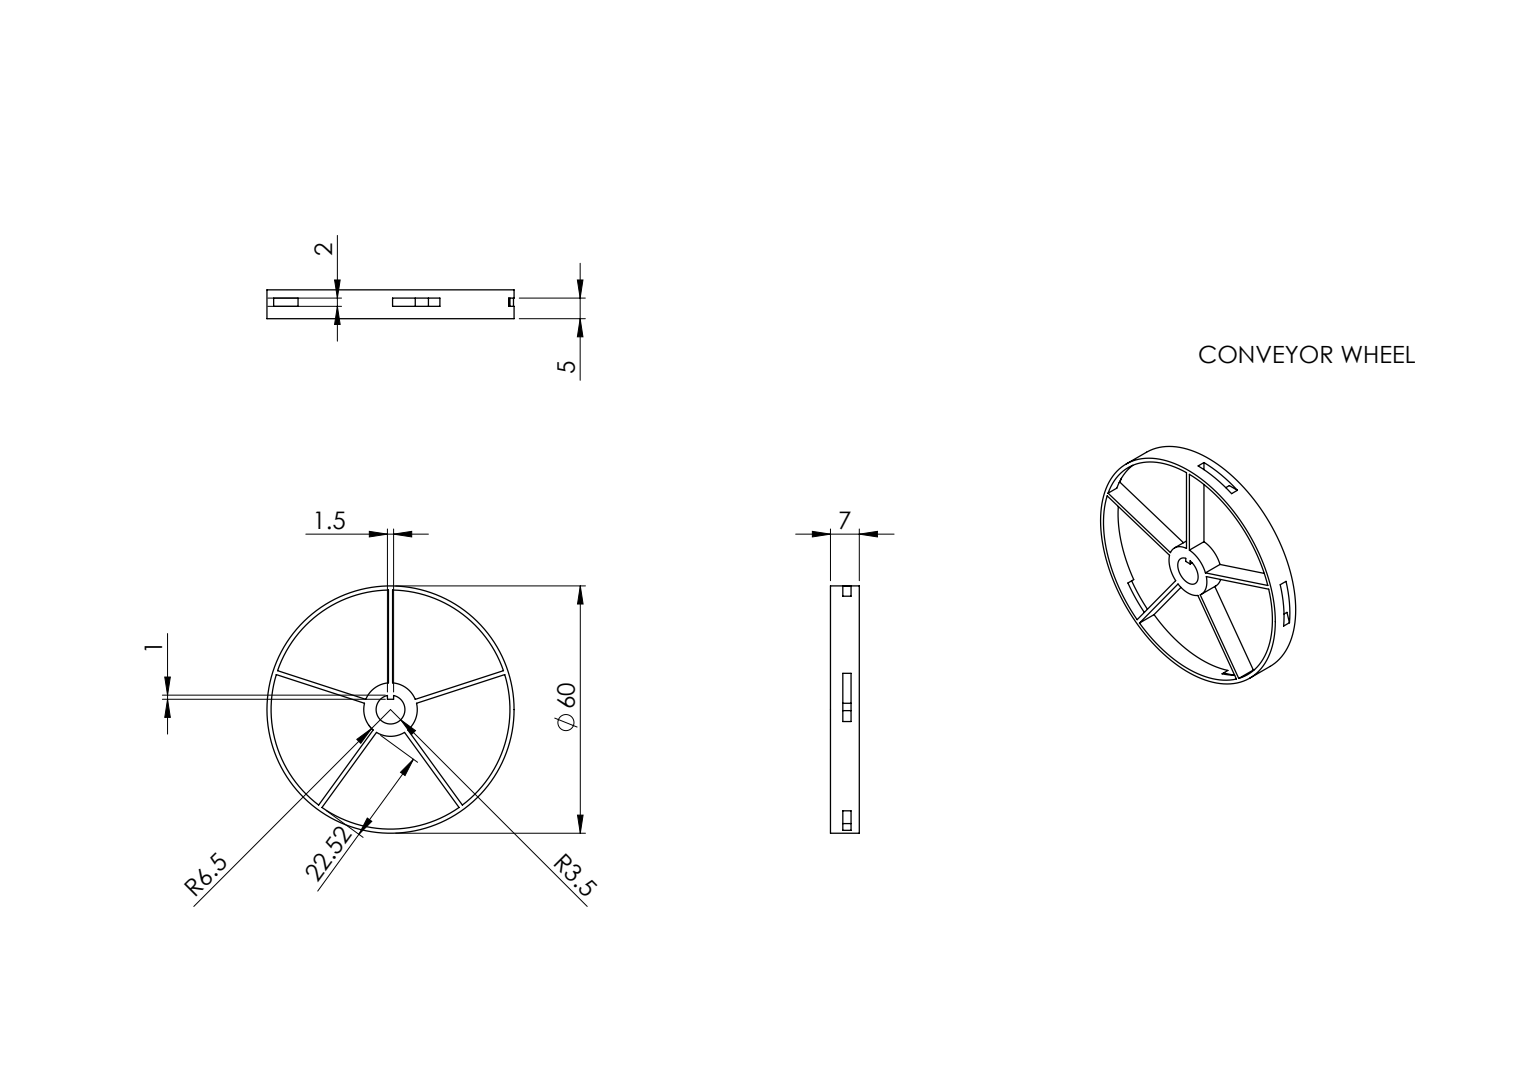
ISO-10303-21;
HEADER;
FILE_DESCRIPTION (('STEP AP214'),
    '1' );
FILE_NAME ('conveyor wheel.step',
    '2026-10-26T05:17:54',
    ( '' ),
    ( '' ),
    'SwSTEP 2.0',
    'SolidWorks 2026',
    '' );
FILE_SCHEMA (( 'AUTOMOTIVE_DESIGN' ));
ENDSEC;

DATA;
#6=FACE_OUTER_BOUND ( 'NONE', #10030, .T. ) ;
#9=CARTESIAN_POINT ( 'NONE',  ( 15.77218708916995560, 135.9950860171967975, 1.000000000000003109 ) ) ;
#22=B_SPLINE_CURVE_WITH_KNOTS ( 'NONE', 3,
 ( #4736, #8602, #10562, #11406 ),
 .UNSPECIFIED., .F., .F.,
 ( 4, 4 ),
 ( 0.000000000000000000, 0.5999999999999992006 ),
 .UNSPECIFIED. ) ;
#23=CARTESIAN_POINT ( 'NONE',  ( 65.00000000000000000, 90.00000000000000000, -3.000000000000000000 ) ) ;
#35=DIRECTION ( 'NONE',  ( -0.000000000000000000, -0.000000000000000000, -1.000000000000000000 ) ) ;
#36=VERTEX_POINT ( 'NONE', #3665 ) ;
#37=LINE ( 'NONE', #7913, #8415 ) ;
#68=ORIENTED_EDGE ( 'NONE', *, *, #7335, .T. ) ;
#69=CARTESIAN_POINT ( 'NONE',  ( 17.26299177799148055, 43.12143982588584379, 1.000000000000003109 ) ) ;
#77=VECTOR ( 'NONE', #7626, 1000.000000000000000 ) ;
#94=CIRCLE ( 'NONE', #5951, 0.9999999999999991118 ) ;
#99=ORIENTED_EDGE ( 'NONE', *, *, #9615, .F. ) ;
#111=FACE_OUTER_BOUND ( 'NONE', #2814, .T. ) ;
#133=LINE ( 'NONE', #6034, #1273 ) ;
#147=ORIENTED_EDGE ( 'NONE', *, *, #622, .F. ) ;
#155=DIRECTION ( 'NONE',  ( -1.000000000000000000, 0.000000000000000000, -0.000000000000000000 ) ) ;
#171=ORIENTED_EDGE ( 'NONE', *, *, #11272, .F. ) ;
#194=CIRCLE ( 'NONE', #6260, 3.499999999999996003 ) ;
#196=ORIENTED_EDGE ( 'NONE', *, *, #12600, .T. ) ;
#199=EDGE_LOOP ( 'NONE', ( #6657, #5220, #2552, #8518 ) ) ;
#210=VECTOR ( 'NONE', #6420, 1000.000000000000000 ) ;
#219=DIRECTION ( 'NONE',  ( 0.000000000000000000, 0.000000000000000000, -1.000000000000000000 ) ) ;
#221=ADVANCED_FACE ( 'NONE', ( #5806 ), #2080, .F. ) ;
#222=PLANE ( 'NONE',  #9692 ) ;
#229=PLANE ( 'NONE',  #10368 ) ;
#233=ORIENTED_EDGE ( 'NONE', *, *, #6025, .F. ) ;
#235=DIRECTION ( 'NONE',  ( -1.000000000000000000, 0.000000000000000000, 0.000000000000000000 ) ) ;
#238=CIRCLE ( 'NONE', #3615, 3.499999999999996003 ) ;
#239=DIRECTION ( 'NONE',  ( 0.000000000000000000, 0.000000000000000000, -1.000000000000000000 ) ) ;
#244=EDGE_CURVE ( 'NONE', #12399, #6272, #479, .T. ) ;
#260=ADVANCED_FACE ( 'NONE', ( #3129 ), #3324, .T. ) ;
#267=CARTESIAN_POINT ( 'NONE',  ( 31.59522469073171891, 84.46307801270442894, 22.38477631085024555 ) ) ;
#274=CARTESIAN_POINT ( 'NONE',  ( 44.20597631976078645, 117.5000000000000568, 4.000000000000000000 ) ) ;
#279=DIRECTION ( 'NONE',  ( -0.5877852522924753575, 0.8090169943749458970, 0.000000000000000000 ) ) ;
#284=AXIS2_PLACEMENT_3D ( 'NONE', #3967, #808, #3834 ) ;
#291=CARTESIAN_POINT ( 'NONE',  ( 35.75000000000000711, 92.49999999999998579, 4.000000000000000000 ) ) ;
#314=LINE ( 'NONE', #2362, #12520 ) ;
#321=DIRECTION ( 'NONE',  ( -0.000000000000000000, -0.000000000000000000, -1.000000000000000000 ) ) ;
#328=ORIENTED_EDGE ( 'NONE', *, *, #4950, .F. ) ;
#330=VERTEX_POINT ( 'NONE', #11158 ) ;
#331=LINE ( 'NONE', #11396, #210 ) ;
#335=ADVANCED_FACE ( 'NONE', ( #1345 ), #222, .F. ) ;
#339=DIRECTION ( 'NONE',  ( -0.5877852522924715828, -0.8090169943749484505, 0.000000000000000000 ) ) ;
#344=CARTESIAN_POINT ( 'NONE',  ( 41.31805916882746743, 91.52713075379783447, 22.38477631085024555 ) ) ;
#348=ORIENTED_EDGE ( 'NONE', *, *, #6229, .T. ) ;
#349=EDGE_CURVE ( 'NONE', #2081, #11940, #2919, .T. ) ;
#352=DIRECTION ( 'NONE',  ( -1.000000000000000000, 0.000000000000000000, 0.000000000000000000 ) ) ;
#353=CARTESIAN_POINT ( 'NONE',  ( 62.42613047537196991, 99.43702109502110886, 4.000000000000000000 ) ) ;
#354=CARTESIAN_POINT ( 'NONE',  ( 17.55170909815984004, 66.83416404266884570, 4.000000000000000000 ) ) ;
#355=ORIENTED_EDGE ( 'NONE', *, *, #8194, .T. ) ;
#356=DIRECTION ( 'NONE',  ( -1.000000000000000000, 0.000000000000000000, 0.000000000000000000 ) ) ;
#363=ORIENTED_EDGE ( 'NONE', *, *, #11341, .T. ) ;
#364=EDGE_CURVE ( 'NONE', #1906, #5411, #4011, .T. ) ;
#371=DIRECTION ( 'NONE',  ( 0.000000000000000000, 0.000000000000000000, -1.000000000000000000 ) ) ;
#372=ORIENTED_EDGE ( 'NONE', *, *, #5978, .T. ) ;
#385=ORIENTED_EDGE ( 'NONE', *, *, #5821, .T. ) ;
#399=CARTESIAN_POINT ( 'NONE',  ( 38.40477530926830951, 84.46307801270444315, -1.000000000000000000 ) ) ;
#413=( LENGTH_UNIT ( ) NAMED_UNIT ( * ) SI_UNIT ( .MILLI., .METRE. ) );
#416=CARTESIAN_POINT ( 'NONE',  ( 35.00000000000000000, 90.00000000000000000, 4.000000000000000000 ) ) ;
#417=CIRCLE ( 'NONE', #3994, 3.499999999999996003 ) ;
#425=CARTESIAN_POINT ( 'NONE',  ( -18.00412335955691745, 88.33754051161746190, 1.000000000000003109 ) ) ;
#429=EDGE_LOOP ( 'NONE', ( #3770, #8264, #6534, #4530, #5902, #2222, #1505, #1439 ) ) ;
#434=ORIENTED_EDGE ( 'NONE', *, *, #4950, .T. ) ;
#440=EDGE_CURVE ( 'NONE', #7916, #8087, #6573, .T. ) ;
#442=CIRCLE ( 'NONE', #5674, 30.00000000000000000 ) ;
#444=CARTESIAN_POINT ( 'NONE',  ( 35.00000000000000000, 90.00000000000000000, 4.000000000000000000 ) ) ;
#454=VERTEX_POINT ( 'NONE', #7693 ) ;
#462=EDGE_CURVE ( 'NONE', #12941, #5885, #2810, .T. ) ;
#465=DIRECTION ( 'NONE',  ( 0.000000000000000000, 0.000000000000000000, -1.000000000000000000 ) ) ;
#467=FACE_OUTER_BOUND ( 'NONE', #11124, .T. ) ;
#470=VECTOR ( 'NONE', #11203, 1000.000000000000000 ) ;
#476=PLANE ( 'NONE',  #4013 ) ;
#479=CIRCLE ( 'NONE', #1327, 28.99999999999999289 ) ;
#491=CARTESIAN_POINT ( 'NONE',  ( 35.00000000000000000, 90.00000000000000000, -0.9999999999999970024 ) ) ;
#493=( GEOMETRIC_REPRESENTATION_CONTEXT ( 3 ) GLOBAL_UNCERTAINTY_ASSIGNED_CONTEXT ( ( #8293 ) ) GLOBAL_UNIT_ASSIGNED_CONTEXT ( ( #12067, #10294, #5125 ) ) REPRESENTATION_CONTEXT ( 'NONE', 'WORKASPACE' ) );
#508=ORIENTED_EDGE ( 'NONE', *, *, #9196, .T. ) ;
#510=ORIENTED_EDGE ( 'NONE', *, *, #7411, .F. ) ;
#512=VECTOR ( 'NONE', #6257, 1000.000000000000000 ) ;
#518=EDGE_LOOP ( 'NONE', ( #12338, #1240, #6550, #7565 ) ) ;
#521=VECTOR ( 'NONE', #8150, 1000.000000000000000 ) ;
#532=CARTESIAN_POINT ( 'NONE',  ( 64.85903780527353035, 87.09520029206045422, -3.000000000000000000 ) ) ;
#536=LINE ( 'NONE', #736, #3548 ) ;
#539=EDGE_CURVE ( 'NONE', #7517, #3017, #9903, .T. ) ;
#566=ORIENTED_EDGE ( 'NONE', *, *, #10069, .F. ) ;
#567=FACE_OUTER_BOUND ( 'NONE', #6153, .T. ) ;
#579=ADVANCED_FACE ( 'NONE', ( #1999 ), #8988, .F. ) ;
#587=VERTEX_POINT ( 'NONE', #749 ) ;
#596=EDGE_CURVE ( 'NONE', #330, #4076, #4069, .T. ) ;
#602=CARTESIAN_POINT ( 'NONE',  ( 35.00000000000000000, 90.00000000000000000, -0.9999999999999970024 ) ) ;
#607=ADVANCED_FACE ( 'NONE', ( #809 ), #12923, .T. ) ;
#610=CARTESIAN_POINT ( 'NONE',  ( 35.00000000000000000, 90.00000000000000000, -1.000000000000000000 ) ) ;
#614=ORIENTED_EDGE ( 'NONE', *, *, #6666, .F. ) ;
#619=VERTEX_POINT ( 'NONE', #8800 ) ;
#622=EDGE_CURVE ( 'NONE', #3150, #9073, #1826, .T. ) ;
#629=ORIENTED_EDGE ( 'NONE', *, *, #7794, .T. ) ;
#630=CARTESIAN_POINT ( 'NONE',  ( 18.35873618070580093, 66.24461453698026503, 4.000000000000000000 ) ) ;
#631=CYLINDRICAL_SURFACE ( 'NONE', #12303, 0.9999999999999991118 ) ;
#663=EDGE_CURVE ( 'NONE', #698, #11775, #6107, .T. ) ;
#665=CARTESIAN_POINT ( 'NONE',  ( 35.00000000000000000, 90.00000000000000000, 4.000000000000000000 ) ) ;
#679=DIRECTION ( 'NONE',  ( 0.9510565162951554186, -0.3090169943749414005, 0.000000000000000000 ) ) ;
#684=COLOUR_RGB ( '',0.8941176470588234615, 0.8941176470588234615, 0.8941176470588234615 ) ;
#698=VERTEX_POINT ( 'NONE', #11012 ) ;
#707=EDGE_CURVE ( 'NONE', #1672, #10599, #4291, .T. ) ;
#726=AXIS2_PLACEMENT_3D ( 'NONE', #602, #12590, #3632 ) ;
#736=CARTESIAN_POINT ( 'NONE',  ( 35.75000000000000711, 92.49999999999998579, -4.802775637732004554 ) ) ;
#737=DIRECTION ( 'NONE',  ( -0.000000000000000000, -0.000000000000000000, -1.000000000000000000 ) ) ;
#745=DIRECTION ( 'NONE',  ( 1.000000000000000000, 1.281026566875180806E-14, 0.000000000000000000 ) ) ;
#749=CARTESIAN_POINT ( 'NONE',  ( 5.000000000000007994, 90.00000000000000000, -3.000000000000000000 ) ) ;
#750=VECTOR ( 'NONE', #11166, 1000.000000000000000 ) ;
#753=DIRECTION ( 'NONE',  ( 1.000000000000000000, 0.000000000000000000, 0.000000000000000000 ) ) ;
#758=ORIENTED_EDGE ( 'NONE', *, *, #6666, .T. ) ;
#772=CARTESIAN_POINT ( 'NONE',  ( 28.99095782554748624, 92.47818727009294548, 4.000000000000000000 ) ) ;
#784=ORIENTED_EDGE ( 'NONE', *, *, #3580, .T. ) ;
#805=PLANE ( 'NONE',  #2672 ) ;
#808=DIRECTION ( 'NONE',  ( -0.000000000000000000, -0.000000000000000000, -1.000000000000000000 ) ) ;
#809=FACE_OUTER_BOUND ( 'NONE', #2682, .T. ) ;
#814=CARTESIAN_POINT ( 'NONE',  ( 28.68194083117252902, 91.52713075379780605, -0.9999999999999970024 ) ) ;
#816=ORIENTED_EDGE ( 'NONE', *, *, #3757, .T. ) ;
#822=DIRECTION ( 'NONE',  ( -0.000000000000000000, -0.000000000000000000, 1.000000000000000000 ) ) ;
#828=CARTESIAN_POINT ( 'NONE',  ( 35.49999999999995026, 119.0000000000000000, 4.000000000000000000 ) ) ;
#838=DIRECTION ( 'NONE',  ( -1.000000000000000000, 0.000000000000000000, 0.000000000000000000 ) ) ;
#851=CARTESIAN_POINT ( 'NONE',  ( 34.25000000000000000, 93.41869858279433458, -3.000000000000000000 ) ) ;
#858=CARTESIAN_POINT ( 'NONE',  ( 51.63879093662676922, 66.24814457421848601, 2.000000000000002220 ) ) ;
#871=AXIS2_PLACEMENT_3D ( 'NONE', #9762, #2644, #10806 ) ;
#889=DIRECTION ( 'NONE',  ( 0.3090169943749451753, 0.9510565162951544194, -0.000000000000000000 ) ) ;
#894=ORIENTED_EDGE ( 'NONE', *, *, #6652, .T. ) ;
#900=ADVANCED_FACE ( 'NONE', ( #10563 ), #6369, .F. ) ;
#901=ORIENTED_EDGE ( 'NONE', *, *, #7854, .T. ) ;
#903=ORIENTED_EDGE ( 'NONE', *, *, #10354, .F. ) ;
#911=AXIS2_PLACEMENT_3D ( 'NONE', #416, #4429, #5462 ) ;
#913=EDGE_CURVE ( 'NONE', #11775, #4019, #4893, .T. ) ;
#924=ORIENTED_EDGE ( 'NONE', *, *, #8530, .F. ) ;
#928=PLANE ( 'NONE',  #5027 ) ;
#940=CARTESIAN_POINT ( 'NONE',  ( 35.00000000000000000, 90.00000000000000000, -1.000000000000000888 ) ) ;
#942=CARTESIAN_POINT ( 'NONE',  ( 39.21379230364324542, 85.05086326499692007, 22.38477631085024555 ) ) ;
#955=VERTEX_POINT ( 'NONE', #7679 ) ;
#967=DIRECTION ( 'NONE',  ( 0.000000000000000000, 0.000000000000000000, -1.000000000000000000 ) ) ;
#970=CIRCLE ( 'NONE', #10176, 28.99999999999999289 ) ;
#984=ORIENTED_EDGE ( 'NONE', *, *, #7294, .F. ) ;
#989=FACE_OUTER_BOUND ( 'NONE', #12469, .T. ) ;
#1002=CIRCLE ( 'NONE', #8121, 28.99999999999999289 ) ;
#1004=EDGE_CURVE ( 'NONE', #6272, #8022, #6754, .T. ) ;
#1018=VERTEX_POINT ( 'NONE', #1792 ) ;
#1029=EDGE_CURVE ( 'NONE', #1627, #698, #2822, .T. ) ;
#1030=EDGE_CURVE ( 'NONE', #9167, #11004, #12112, .T. ) ;
#1035=ORIENTED_EDGE ( 'NONE', *, *, #1030, .F. ) ;
#1047=CARTESIAN_POINT ( 'NONE',  ( 34.49999999999995026, 119.0000000000000000, 4.000000000000000000 ) ) ;
#1053=LINE ( 'NONE', #12841, #6033 ) ;
#1055=EDGE_LOOP ( 'NONE', ( #6384, #2925 ) ) ;
#1065=CARTESIAN_POINT ( 'NONE',  ( 11.38811426945698635, 73.16316976839823383, 1.000000000000003109 ) ) ;
#1068=CARTESIAN_POINT ( 'NONE',  ( 17.54971918633085437, 66.83239978927272773, 4.000000000000000000 ) ) ;
#1093=DIRECTION ( 'NONE',  ( 0.9510565162951530871, 0.3090169943749492276, 0.000000000000000000 ) ) ;
#1112=ADVANCED_FACE ( 'NONE', ( #1366, #12361, #1118 ), #3474, .T. ) ;
#1114=ORIENTED_EDGE ( 'NONE', *, *, #12529, .F. ) ;
#1118=FACE_BOUND ( 'NONE', #9389, .T. ) ;
#1120=EDGE_CURVE ( 'NONE', #11429, #7517, #11126, .T. ) ;
#1121=VECTOR ( 'NONE', #8149, 1000.000000000000000 ) ;
#1132=DIRECTION ( 'NONE',  ( -1.000000000000000000, 0.000000000000000000, 0.000000000000000000 ) ) ;
#1165=ORIENTED_EDGE ( 'NONE', *, *, #10513, .T. ) ;
#1172=CIRCLE ( 'NONE', #3276, 3.499999999999996003 ) ;
#1174=DIRECTION ( 'NONE',  ( 1.000000000000000000, 0.000000000000000000, -0.000000000000000000 ) ) ;
#1176=ORIENTED_EDGE ( 'NONE', *, *, #9094, .T. ) ;
#1191=VECTOR ( 'NONE', #4790, 1000.000000000000227 ) ;
#1197=CARTESIAN_POINT ( 'NONE',  ( 62.42613047537196991, 99.43702109502110886, -1.000000000000000000 ) ) ;
#1199=DIRECTION ( 'NONE',  ( -0.000000000000000000, -0.000000000000000000, -1.000000000000000000 ) ) ;
#1202=CARTESIAN_POINT ( 'NONE',  ( 35.75000000000000711, 93.41869858279433458, 4.000000000000000000 ) ) ;
#1203=CARTESIAN_POINT ( 'NONE',  ( 35.00000000000000000, 90.00000000000000000, 4.000000000000000000 ) ) ;
#1204=CARTESIAN_POINT ( 'NONE',  ( 34.49999999999995026, 119.0000000000000000, -1.000000000000000000 ) ) ;
#1218=AXIS2_PLACEMENT_3D ( 'NONE', #11961, #967, #235 ) ;
#1224=VERTEX_POINT ( 'NONE', #5684 ) ;
#1225=CARTESIAN_POINT ( 'NONE',  ( 34.25000000000000000, 93.50000000000000000, -4.802775637732004554 ) ) ;
#1232=PRODUCT_DEFINITION_CONTEXT ( 'detailed design', #12541, 'design' ) ;
#1240=ORIENTED_EDGE ( 'NONE', *, *, #11905, .F. ) ;
#1241=APPLICATION_CONTEXT ( 'automotive_design' ) ;
#1250=EDGE_CURVE ( 'NONE', #8496, #7310, #9672, .T. ) ;
#1255=CARTESIAN_POINT ( 'NONE',  ( 34.25000000000000000, 92.49999999999998579, -3.000000000000000000 ) ) ;
#1268=CYLINDRICAL_SURFACE ( 'NONE', #7741, 28.99999999999999289 ) ;
#1273=VECTOR ( 'NONE', #9896, 1000.000000000000000 ) ;
#1278=VERTEX_POINT ( 'NONE', #4514 ) ;
#1280=AXIS2_PLACEMENT_3D ( 'NONE', #7330, #12243, #1438 ) ;
#1281=CARTESIAN_POINT ( 'NONE',  ( 51.64126381929429499, 66.24461453698036451, -1.000000000000000000 ) ) ;
#1315=ORIENTED_EDGE ( 'NONE', *, *, #9075, .F. ) ;
#1320=AXIS2_PLACEMENT_3D ( 'NONE', #7964, #5805, #9918 ) ;
#1324=CARTESIAN_POINT ( 'NONE',  ( 35.00000000000000000, 90.00000000000000000, 4.000000000000000000 ) ) ;
#1327=AXIS2_PLACEMENT_3D ( 'NONE', #5273, #7305, #8292 ) ;
#1336=DIRECTION ( 'NONE',  ( 0.000000000000000000, 0.000000000000000000, -1.000000000000000000 ) ) ;
#1338=VECTOR ( 'NONE', #6044, 1000.000000000000000 ) ;
#1345=FACE_OUTER_BOUND ( 'NONE', #11526, .T. ) ;
#1349=DIRECTION ( 'NONE',  ( 0.000000000000000000, 0.000000000000000000, -1.000000000000000000 ) ) ;
#1366=FACE_OUTER_BOUND ( 'NONE', #429, .T. ) ;
#1378=ORIENTED_EDGE ( 'NONE', *, *, #3459, .T. ) ;
#1388=CARTESIAN_POINT ( 'NONE',  ( 35.00000000000000000, 90.00000000000000000, -1.000000000000000888 ) ) ;
#1395=ADVANCED_FACE ( 'NONE', ( #7838 ), #9861, .F. ) ;
#1400=CIRCLE ( 'NONE', #8716, 6.499999999999999112 ) ;
#1402=CARTESIAN_POINT ( 'NONE',  ( 35.00000000000000000, 90.00000000000000000, -1.000000000000000000 ) ) ;
#1404=ORIENTED_EDGE ( 'NONE', *, *, #12529, .T. ) ;
#1417=EDGE_LOOP ( 'NONE', ( #9875, #11327, #1315, #8579, #2320, #12149 ) ) ;
#1418=CARTESIAN_POINT ( 'NONE',  ( 35.00000000000000000, 90.00000000000000000, -3.000000000000000000 ) ) ;
#1438=DIRECTION ( 'NONE',  ( -1.000000000000000000, 0.000000000000000000, 0.000000000000000000 ) ) ;
#1439=ORIENTED_EDGE ( 'NONE', *, *, #2364, .F. ) ;
#1441=LINE ( 'NONE', #3416, #7058 ) ;
#1460=CARTESIAN_POINT ( 'NONE',  ( 9.136132550659258555, 74.79933025939540414, -3.000000000000000000 ) ) ;
#1462=DIRECTION ( 'NONE',  ( -0.000000000000000000, -0.000000000000000000, -1.000000000000000000 ) ) ;
#1477=CARTESIAN_POINT ( 'NONE',  ( 35.49951382533862443, 118.9974510565036070, 4.000000000000000000 ) ) ;
#1497=VERTEX_POINT ( 'NONE', #1822 ) ;
#1499=EDGE_LOOP ( 'NONE', ( #11671, #99, #12405, #1707, #12220, #9341 ) ) ;
#1502=ORIENTED_EDGE ( 'NONE', *, *, #8330, .T. ) ;
#1505=ORIENTED_EDGE ( 'NONE', *, *, #9242, .T. ) ;
#1518=EDGE_CURVE ( 'NONE', #619, #8102, #2838, .T. ) ;
#1523=LINE ( 'NONE', #8338, #7931 ) ;
#1524=EDGE_CURVE ( 'NONE', #8087, #11248, #2282, .T. ) ;
#1535=EDGE_LOOP ( 'NONE', ( #6310, #2117, #8009, #1866 ) ) ;
#1537=DIRECTION ( 'NONE',  ( -1.000000000000000000, 0.000000000000000000, 0.000000000000000000 ) ) ;
#1549=DIRECTION ( 'NONE',  ( -1.000000000000000000, 0.000000000000000000, -0.000000000000000000 ) ) ;
#1573=VECTOR ( 'NONE', #371, 1000.000000000000000 ) ;
#1585=VERTEX_POINT ( 'NONE', #8295 ) ;
#1591=AXIS2_PLACEMENT_3D ( 'NONE', #9703, #4864, #1793 ) ;
#1593=CIRCLE ( 'NONE', #8488, 30.00000000000000000 ) ;
#1597=CARTESIAN_POINT ( 'NONE',  ( 64.99999999999998579, 122.5000000000001847, 1.000000000000003109 ) ) ;
#1598=DIRECTION ( 'NONE',  ( -1.914177628664063178E-15, 1.000000000000000000, 0.000000000000000000 ) ) ;
#1600=VECTOR ( 'NONE', #11685, 1000.000000000000000 ) ;
#1618=DIRECTION ( 'NONE',  ( -1.000000000000000000, 0.000000000000000000, 0.000000000000000000 ) ) ;
#1620=CIRCLE ( 'NONE', #5170, 28.99999999999999289 ) ;
#1627=VERTEX_POINT ( 'NONE', #10313 ) ;
#1638=ORIENTED_EDGE ( 'NONE', *, *, #11170, .F. ) ;
#1643=UNCERTAINTY_MEASURE_WITH_UNIT (LENGTH_MEASURE( 1.000000000000000082E-05 ), #413, 'distance_accuracy_value', 'NONE');
#1647=DIRECTION ( 'NONE',  ( 0.8090169943749456749, -0.5877852522924754686, 0.000000000000000000 ) ) ;
#1655=DIRECTION ( 'NONE',  ( -1.000000000000000000, 0.000000000000000000, 0.000000000000000000 ) ) ;
#1664=DIRECTION ( 'NONE',  ( 0.9510565162951543083, -0.3090169943749451198, 0.000000000000000000 ) ) ;
#1672=VERTEX_POINT ( 'NONE', #4242 ) ;
#1686=ORIENTED_EDGE ( 'NONE', *, *, #3091, .T. ) ;
#1688=DIRECTION ( 'NONE',  ( 0.5877852522924715828, 0.8090169943749485615, 0.000000000000000000 ) ) ;
#1707=ORIENTED_EDGE ( 'NONE', *, *, #2445, .T. ) ;
#1726=CARTESIAN_POINT ( 'NONE',  ( 18.35873618070580093, 66.24461453698026503, 2.333333333333333481 ) ) ;
#1748=CYLINDRICAL_SURFACE ( 'NONE', #6951, 28.99999999999999289 ) ;
#1750=CARTESIAN_POINT ( 'NONE',  ( 35.00000000000000000, 90.00000000000000000, 22.38477631085024555 ) ) ;
#1759=ORIENTED_EDGE ( 'NONE', *, *, #6632, .F. ) ;
#1773=EDGE_LOOP ( 'NONE', ( #4370, #8040, #4865, #4151 ) ) ;
#1783=DIRECTION ( 'NONE',  ( 0.000000000000000000, 0.000000000000000000, 1.000000000000000000 ) ) ;
#1791=FACE_BOUND ( 'NONE', #2135, .T. ) ;
#1792=CARTESIAN_POINT ( 'NONE',  ( 39.21379230364325252, 85.05086326499692007, 4.000000000000000000 ) ) ;
#1793=DIRECTION ( 'NONE',  ( -1.000000000000000000, 0.000000000000000000, 0.000000000000000000 ) ) ;
#1805=DIRECTION ( 'NONE',  ( 1.000000000000000000, 0.000000000000000000, 0.000000000000000000 ) ) ;
#1811=DIRECTION ( 'NONE',  ( -1.000000000000000000, 0.000000000000000000, 0.000000000000000000 ) ) ;
#1822=CARTESIAN_POINT ( 'NONE',  ( 44.20597631976078645, 117.5000000000000568, -0.9999999999999974465 ) ) ;
#1826=B_SPLINE_CURVE_WITH_KNOTS ( 'NONE', 3,
 ( #8864, #11935, #9844, #3836 ),
 .UNSPECIFIED., .F., .F.,
 ( 4, 4 ),
 ( 0.000000000000000000, 1.000000000000000000 ),
 .UNSPECIFIED. ) ;
#1832=DIRECTION ( 'NONE',  ( 0.000000000000000000, 0.000000000000000000, 1.000000000000000000 ) ) ;
#1839=EDGE_CURVE ( 'NONE', #12641, #8130, #11823, .T. ) ;
#1853=CARTESIAN_POINT ( 'NONE',  ( 43.71630314554308683, 62.34089554097972297, 4.000000000000000000 ) ) ;
#1855=CARTESIAN_POINT ( 'NONE',  ( 51.63879093662676922, 66.24814457421848601, 3.000000000000000888 ) ) ;
#1857=CARTESIAN_POINT ( 'NONE',  ( 13.22666678878058200, 110.6378768499380527, 1.000000000000003553 ) ) ;
#1866=ORIENTED_EDGE ( 'NONE', *, *, #1004, .F. ) ;
#1868=CARTESIAN_POINT ( 'NONE',  ( 34.50001867552290946, 118.9978264099154615, 4.000000000000000000 ) ) ;
#1869=CARTESIAN_POINT ( 'NONE',  ( 35.00000000000000000, 90.00000000000000000, 1.000000000000003553 ) ) ;
#1889=ORIENTED_EDGE ( 'NONE', *, *, #9910, .T. ) ;
#1893=DIRECTION ( 'NONE',  ( -1.000000000000000000, -3.349810850162111054E-15, 0.000000000000000000 ) ) ;
#1896=AXIS2_PLACEMENT_3D ( 'NONE', #6709, #8681, #753 ) ;
#1899=DIRECTION ( 'NONE',  ( -1.000000000000000000, 0.000000000000000000, 0.000000000000000000 ) ) ;
#1906=VERTEX_POINT ( 'NONE', #9783 ) ;
#1931=CARTESIAN_POINT ( 'NONE',  ( 35.00000000000000000, 90.00000000000000000, 1.000000000000003553 ) ) ;
#1961=ORIENTED_EDGE ( 'NONE', *, *, #5470, .T. ) ;
#1976=VECTOR ( 'NONE', #2128, 1000.000000000000000 ) ;
#1979=EDGE_CURVE ( 'NONE', #8306, #6159, #5913, .T. ) ;
#1995=EDGE_CURVE ( 'NONE', #10403, #1497, #9321, .T. ) ;
#1998=CARTESIAN_POINT ( 'NONE',  ( 28.68194083117254323, 91.52713075379780605, 4.000000000000000000 ) ) ;
#1999=FACE_OUTER_BOUND ( 'NONE', #11000, .T. ) ;
#2007=ORIENTED_EDGE ( 'NONE', *, *, #3459, .F. ) ;
#2012=LINE ( 'NONE', #6974, #4777 ) ;
#2013=DIRECTION ( 'NONE',  ( 0.8090169943749476733, 0.5877852522924726930, 0.000000000000000000 ) ) ;
#2029=ORIENTED_EDGE ( 'NONE', *, *, #3482, .T. ) ;
#2048=CARTESIAN_POINT ( 'NONE',  ( 62.73303611935715196, 98.48533184915085315, 4.000000000000000000 ) ) ;
#2051=ORIENTED_EDGE ( 'NONE', *, *, #4067, .T. ) ;
#2067=VECTOR ( 'NONE', #1199, 1000.000000000000000 ) ;
#2070=ORIENTED_EDGE ( 'NONE', *, *, #6607, .T. ) ;
#2072=ORIENTED_EDGE ( 'NONE', *, *, #4557, .F. ) ;
#2080=PLANE ( 'NONE',  #9893 ) ;
#2081=VERTEX_POINT ( 'NONE', #10100 ) ;
#2117=ORIENTED_EDGE ( 'NONE', *, *, #10147, .T. ) ;
#2120=LINE ( 'NONE', #9835, #10672 ) ;
#2128=DIRECTION ( 'NONE',  ( 0.000000000000000000, 0.000000000000000000, 1.000000000000000000 ) ) ;
#2135=EDGE_LOOP ( 'NONE', ( #6787, #2219, #4205, #4367, #1961, #1404 ) ) ;
#2158=CARTESIAN_POINT ( 'NONE',  ( 13.22666678878058200, 110.6378768499380527, -1.000000000000000000 ) ) ;
#2171=CARTESIAN_POINT ( 'NONE',  ( 34.25000000000000000, 93.41869858279433458, 22.38477631085024555 ) ) ;
#2187=AXIS2_PLACEMENT_3D ( 'NONE', #1931, #9118, #1132 ) ;
#2189=CARTESIAN_POINT ( 'NONE',  ( 62.42406877824604550, 99.43633191144624561, -1.000000000000000222 ) ) ;
#2194=CARTESIAN_POINT ( 'NONE',  ( 63.99885733073619321, 89.74256357754357794, 4.000000000000000000 ) ) ;
#2203=AXIS2_PLACEMENT_3D ( 'NONE', #9334, #8226, #356 ) ;
#2215=VECTOR ( 'NONE', #9482, 1000.000000000000000 ) ;
#2218=CARTESIAN_POINT ( 'NONE',  ( 30.78620769635677235, 85.05086326499690585, 22.38477631085024555 ) ) ;
#2219=ORIENTED_EDGE ( 'NONE', *, *, #10889, .F. ) ;
#2221=CARTESIAN_POINT ( 'NONE',  ( 63.68224097532933570, 98.79369391286385849, -3.000000000000000000 ) ) ;
#2222=ORIENTED_EDGE ( 'NONE', *, *, #596, .F. ) ;
#2241=EDGE_CURVE ( 'NONE', #12941, #11688, #2718, .T. ) ;
#2245=DIRECTION ( 'NONE',  ( 1.914177628664063178E-15, -1.000000000000000000, 0.000000000000000000 ) ) ;
#2258=EDGE_CURVE ( 'NONE', #4025, #3338, #5451, .T. ) ;
#2272=ORIENTED_EDGE ( 'NONE', *, *, #3616, .F. ) ;
#2274=CARTESIAN_POINT ( 'NONE',  ( 52.45028081366923089, 66.83239978927284142, 4.000000000000000000 ) ) ;
#2279=CARTESIAN_POINT ( 'NONE',  ( 52.45028081366923089, 66.83239978927284142, 4.000000000000000000 ) ) ;
#2282=LINE ( 'NONE', #291, #512 ) ;
#2288=ORIENTED_EDGE ( 'NONE', *, *, #1004, .T. ) ;
#2290=VECTOR ( 'NONE', #5580, 1000.000000000000000 ) ;
#2304=DIRECTION ( 'NONE',  ( -1.000000000000000000, -5.551115123125781124E-15, 0.000000000000000000 ) ) ;
#2305=ORIENTED_EDGE ( 'NONE', *, *, #12144, .T. ) ;
#2319=LINE ( 'NONE', #6030, #470 ) ;
#2320=ORIENTED_EDGE ( 'NONE', *, *, #7949, .F. ) ;
#2323=ADVANCED_FACE ( 'NONE', ( #7019 ), #4804, .T. ) ;
#2328=DIRECTION ( 'NONE',  ( -1.000000000000000000, 0.000000000000000000, 0.000000000000000000 ) ) ;
#2362=CARTESIAN_POINT ( 'NONE',  ( 34.49999999999998579, 96.48074069840785683, 22.38477631085024555 ) ) ;
#2364=EDGE_CURVE ( 'NONE', #6336, #8478, #7652, .T. ) ;
#2365=CARTESIAN_POINT ( 'NONE',  ( 38.50000000000000000, 90.00000000000000000, -3.000000000000000000 ) ) ;
#2366=EDGE_CURVE ( 'NONE', #10005, #8267, #6599, .T. ) ;
#2369=DIRECTION ( 'NONE',  ( -0.5877852522924710277, 0.8090169943749490056, 0.000000000000000000 ) ) ;
#2374=ORIENTED_EDGE ( 'NONE', *, *, #8330, .F. ) ;
#2387=CARTESIAN_POINT ( 'NONE',  ( 41.00904217445251732, 92.47818727009297390, 22.38477631085024555 ) ) ;
#2394=DIRECTION ( 'NONE',  ( 1.000000000000000000, 2.135044278125301343E-15, 0.000000000000000000 ) ) ;
#2403=LINE ( 'NONE', #5775, #8274 ) ;
#2411=AXIS2_PLACEMENT_3D ( 'NONE', #1068, #9183, #339 ) ;
#2413=DIRECTION ( 'NONE',  ( -1.000000000000000000, 0.000000000000000000, 0.000000000000000000 ) ) ;
#2414=ORIENTED_EDGE ( 'NONE', *, *, #10673, .T. ) ;
#2445=EDGE_CURVE ( 'NONE', #11236, #5069, #2909, .T. ) ;
#2453=CARTESIAN_POINT ( 'NONE',  ( 7.573869524628007888, 99.43702109502098097, 4.000000000000000000 ) ) ;
#2455=EDGE_CURVE ( 'NONE', #8074, #6272, #11131, .T. ) ;
#2456=DIRECTION ( 'NONE',  ( -1.000000000000000000, 0.000000000000000000, -0.000000000000000000 ) ) ;
#2467=( NAMED_UNIT ( * ) PLANE_ANGLE_UNIT ( ) SI_UNIT ( $, .RADIAN. ) );
#2475=ORIENTED_EDGE ( 'NONE', *, *, #7794, .F. ) ;
#2491=SHAPE_DEFINITION_REPRESENTATION ( #6355, #7342 ) ;
#2511=AXIS2_PLACEMENT_3D ( 'NONE', #6884, #5777, #9767 ) ;
#2512=CARTESIAN_POINT ( 'NONE',  ( 64.85903780527353035, 87.09520029206045422, 1.000000000000003553 ) ) ;
#2519=VECTOR ( 'NONE', #1349, 1000.000000000000000 ) ;
#2525=CARTESIAN_POINT ( 'NONE',  ( 35.00000000000000000, 90.00000000000000000, 4.000000000000000000 ) ) ;
#2540=ORIENTED_EDGE ( 'NONE', *, *, #11563, .T. ) ;
#2542=ORIENTED_EDGE ( 'NONE', *, *, #349, .F. ) ;
#2551=CARTESIAN_POINT ( 'NONE',  ( 35.00000000000000000, 90.00000000000000000, -0.9999999999999970024 ) ) ;
#2552=ORIENTED_EDGE ( 'NONE', *, *, #8701, .F. ) ;
#2562=CARTESIAN_POINT ( 'NONE',  ( 35.00000000000000000, 90.00000000000000000, -1.000000000000000000 ) ) ;
#2572=ORIENTED_EDGE ( 'NONE', *, *, #12077, .T. ) ;
#2575=CARTESIAN_POINT ( 'NONE',  ( 35.00000000000000000, 90.00000000000000000, 4.000000000000000000 ) ) ;
#2576=FACE_OUTER_BOUND ( 'NONE', #10821, .T. ) ;
#2579=STYLED_ITEM ( 'NONE', ( #11547 ), #9016 ) ;
#2592=ORIENTED_EDGE ( 'NONE', *, *, #7347, .F. ) ;
#2598=EDGE_CURVE ( 'NONE', #1585, #3338, #2319, .T. ) ;
#2601=EDGE_LOOP ( 'NONE', ( #4533, #2070, #7751, #6048 ) ) ;
#2613=AXIS2_PLACEMENT_3D ( 'NONE', #8406, #9578, #12389 ) ;
#2618=DIRECTION ( 'NONE',  ( 0.8090169943749456749, -0.5877852522924754686, 0.000000000000000000 ) ) ;
#2631=EDGE_LOOP ( 'NONE', ( #8821, #12095, #8765, #147 ) ) ;
#2635=PLANE ( 'NONE',  #6877 ) ;
#2644=DIRECTION ( 'NONE',  ( 0.9510565162951528650, 0.3090169943749500048, 0.000000000000000000 ) ) ;
#2649=CARTESIAN_POINT ( 'NONE',  ( 52.45028081366923089, 66.83239978927284142, -1.000000000000000000 ) ) ;
#2650=CYLINDRICAL_SURFACE ( 'NONE', #8253, 3.499999999999996003 ) ;
#2664=ADVANCED_FACE ( 'NONE', ( #5766, #10068, #4131, #7131, #4261, #8118, #10135 ), #11184, .T. ) ;
#2669=FACE_OUTER_BOUND ( 'NONE', #1773, .T. ) ;
#2672=AXIS2_PLACEMENT_3D ( 'NONE', #5721, #7947, #2977 ) ;
#2681=DIRECTION ( 'NONE',  ( -1.914177628664063178E-15, 1.000000000000000000, 0.000000000000000000 ) ) ;
#2682=EDGE_LOOP ( 'NONE', ( #9674, #629, #7586, #5744 ) ) ;
#2686=B_SPLINE_CURVE_WITH_KNOTS ( 'NONE', 3,
 ( #10985, #6874, #10072, #8963 ),
 .UNSPECIFIED., .F., .F.,
 ( 4, 4 ),
 ( 0.000000000000000000, 0.5999999999999995337 ),
 .UNSPECIFIED. ) ;
#2694=CARTESIAN_POINT ( 'NONE',  ( 35.49999999999999289, 96.48074069840785683, 4.000000000000000000 ) ) ;
#2716=CARTESIAN_POINT ( 'NONE',  ( 18.35873618070580093, 66.24461453698026503, 0.6666666666666665186 ) ) ;
#2718=LINE ( 'NONE', #6564, #9099 ) ;
#2728=CARTESIAN_POINT ( 'NONE',  ( 35.00000000000000000, 90.00000000000000000, 4.000000000000000000 ) ) ;
#2742=AXIS2_PLACEMENT_3D ( 'NONE', #5574, #12709, #9691 ) ;
#2743=CARTESIAN_POINT ( 'NONE',  ( 35.75000000000000711, 92.49999999999998579, -3.000000000000000000 ) ) ;
#2746=CARTESIAN_POINT ( 'NONE',  ( 34.50001850811341342, 118.9978265420697170, -1.000000000000000000 ) ) ;
#2753=AXIS2_PLACEMENT_3D ( 'NONE', #7733, #8779, #10616 ) ;
#2760=AXIS2_PLACEMENT_3D ( 'NONE', #444, #11769, #1893 ) ;
#2773=CIRCLE ( 'NONE', #7992, 28.99999999999999289 ) ;
#2788=( NAMED_UNIT ( * ) SI_UNIT ( $, .STERADIAN. ) SOLID_ANGLE_UNIT ( ) );
#2789=( GEOMETRIC_REPRESENTATION_CONTEXT ( 3 ) GLOBAL_UNCERTAINTY_ASSIGNED_CONTEXT ( ( #1643 ) ) GLOBAL_UNIT_ASSIGNED_CONTEXT ( ( #413, #2467, #6441 ) ) REPRESENTATION_CONTEXT ( 'NONE', 'WORKASPACE' ) );
#2798=LINE ( 'NONE', #4037, #3708 ) ;
#2803=EDGE_CURVE ( 'NONE', #698, #4148, #11946, .T. ) ;
#2810=CIRCLE ( 'NONE', #911, 3.499999999999996003 ) ;
#2814=EDGE_LOOP ( 'NONE', ( #12536, #11570, #363, #2374, #3035 ) ) ;
#2820=CARTESIAN_POINT ( 'NONE',  ( 35.00000000000000000, 90.00000000000000000, -3.000000000000000000 ) ) ;
#2822=CIRCLE ( 'NONE', #4285, 29.99999999999999645 ) ;
#2823=CIRCLE ( 'NONE', #726, 30.00000000000000000 ) ;
#2831=ORIENTED_EDGE ( 'NONE', *, *, #11272, .T. ) ;
#2834=CARTESIAN_POINT ( 'NONE',  ( 35.00000000000000000, 90.00000000000000000, 1.000000000000003109 ) ) ;
#2837=EDGE_CURVE ( 'NONE', #7663, #9298, #12615, .T. ) ;
#2838=CIRCLE ( 'NONE', #2203, 28.99999999999999289 ) ;
#2844=DIRECTION ( 'NONE',  ( 0.000000000000000000, 0.000000000000000000, -1.000000000000000000 ) ) ;
#2846=CARTESIAN_POINT ( 'NONE',  ( 66.06384527677998619, 99.56752405903819181, 1.000000000000003109 ) ) ;
#2871=CARTESIAN_POINT ( 'NONE',  ( 11.38811426945699345, 73.16316976839823383, -0.9999999999999970024 ) ) ;
#2877=CARTESIAN_POINT ( 'NONE',  ( 7.573869524628007888, 99.43702109502098097, -1.000000000000000000 ) ) ;
#2888=ORIENTED_EDGE ( 'NONE', *, *, #3152, .F. ) ;
#2889=LINE ( 'NONE', #6674, #8057 ) ;
#2899=CARTESIAN_POINT ( 'NONE',  ( 35.49999999999994316, 119.9958330439412890, 1.000000000000003109 ) ) ;
#2909=LINE ( 'NONE', #2846, #8897 ) ;
#2919=B_SPLINE_CURVE_WITH_KNOTS ( 'NONE', 3,
 ( #354, #5142, #10181, #4365 ),
 .UNSPECIFIED., .F., .F.,
 ( 4, 4 ),
 ( 0.000000000000000000, 0.5999999999999994227 ),
 .UNSPECIFIED. ) ;
#2925=ORIENTED_EDGE ( 'NONE', *, *, #2364, .T. ) ;
#2927=CIRCLE ( 'NONE', #10231, 6.499999999999999112 ) ;
#2928=CARTESIAN_POINT ( 'NONE',  ( 62.42406877824604550, 99.43633191144624561, -1.000000000000000222 ) ) ;
#2930=EDGE_CURVE ( 'NONE', #6279, #8102, #11826, .T. ) ;
#2953=ORIENTED_EDGE ( 'NONE', *, *, #11170, .T. ) ;
#2966=ADVANCED_FACE ( 'NONE', ( #11157 ), #3262, .F. ) ;
#2977=DIRECTION ( 'NONE',  ( -1.000000000000000000, 0.000000000000000000, -0.000000000000000000 ) ) ;
#2985=EDGE_LOOP ( 'NONE', ( #9465, #9544, #12255, #9850 ) ) ;
#3000=ORIENTED_EDGE ( 'NONE', *, *, #5978, .F. ) ;
#3006=FACE_OUTER_BOUND ( 'NONE', #11503, .T. ) ;
#3011=ORIENTED_EDGE ( 'NONE', *, *, #3949, .T. ) ;
#3017=VERTEX_POINT ( 'NONE', #11224 ) ;
#3025=CARTESIAN_POINT ( 'NONE',  ( 7.264852530253062213, 98.48596457872582732, -1.000000000000000000 ) ) ;
#3026=EDGE_CURVE ( 'NONE', #4743, #12641, #3062, .T. ) ;
#3030=DIRECTION ( 'NONE',  ( -1.000000000000000000, 0.000000000000000000, 0.000000000000000000 ) ) ;
#3032=ORIENTED_EDGE ( 'NONE', *, *, #10147, .F. ) ;
#3035=ORIENTED_EDGE ( 'NONE', *, *, #2445, .F. ) ;
#3047=CYLINDRICAL_SURFACE ( 'NONE', #284, 3.499999999999996003 ) ;
#3054=LINE ( 'NONE', #7036, #8289 ) ;
#3058=ORIENTED_EDGE ( 'NONE', *, *, #10619, .F. ) ;
#3061=DIRECTION ( 'NONE',  ( -0.000000000000000000, -0.000000000000000000, -1.000000000000000000 ) ) ;
#3062=LINE ( 'NONE', #5140, #11403 ) ;
#3065=DIRECTION ( 'NONE',  ( -0.9510565162951543083, 0.3090169943749451198, 0.000000000000000000 ) ) ;
#3070=PLANE ( 'NONE',  #9530 ) ;
#3076=PLANE ( 'NONE',  #10502 ) ;
#3087=DIRECTION ( 'NONE',  ( 0.000000000000000000, 0.000000000000000000, 1.000000000000000000 ) ) ;
#3091=EDGE_CURVE ( 'NONE', #4148, #4871, #9456, .T. ) ;
#3092=AXIS2_PLACEMENT_3D ( 'NONE', #11807, #7750, #745 ) ;
#3100=DIRECTION ( 'NONE',  ( 1.000000000000000000, 0.000000000000000000, 0.000000000000000000 ) ) ;
#3102=EDGE_LOOP ( 'NONE', ( #385, #5025 ) ) ;
#3107=EDGE_LOOP ( 'NONE', ( #901, #816, #9398, #233 ) ) ;
#3129=FACE_OUTER_BOUND ( 'NONE', #9879, .T. ) ;
#3139=DIRECTION ( 'NONE',  ( 0.000000000000000000, 0.000000000000000000, 1.000000000000000000 ) ) ;
#3150=VERTEX_POINT ( 'NONE', #5396 ) ;
#3152=EDGE_CURVE ( 'NONE', #8914, #6886, #2403, .T. ) ;
#3153=DIRECTION ( 'NONE',  ( 0.000000000000000000, 0.000000000000000000, 1.000000000000000000 ) ) ;
#3172=DIRECTION ( 'NONE',  ( 0.000000000000000000, -1.000000000000000000, 0.000000000000000000 ) ) ;
#3211=MECHANICAL_DESIGN_GEOMETRIC_PRESENTATION_REPRESENTATION('',(#2579),#12619);
#3225=VECTOR ( 'NONE', #9394, 1000.000000000000000 ) ;
#3243=LINE ( 'NONE', #1197, #4348 ) ;
#3251=DIRECTION ( 'NONE',  ( 0.000000000000000000, 0.000000000000000000, 1.000000000000000000 ) ) ;
#3262=PLANE ( 'NONE',  #11349 ) ;
#3269=CARTESIAN_POINT ( 'NONE',  ( 41.31805916882746033, 91.52713075379783447, -1.000000000000000000 ) ) ;
#3276=AXIS2_PLACEMENT_3D ( 'NONE', #1418, #10641, #1618 ) ;
#3287=EDGE_LOOP ( 'NONE', ( #508, #7957, #6808, #12755 ) ) ;
#3290=DIRECTION ( 'NONE',  ( 0.000000000000000000, 0.000000000000000000, 1.000000000000000000 ) ) ;
#3295=ORIENTED_EDGE ( 'NONE', *, *, #10929, .F. ) ;
#3301=EDGE_CURVE ( 'NONE', #587, #6336, #5487, .T. ) ;
#3320=ORIENTED_EDGE ( 'NONE', *, *, #3554, .T. ) ;
#3324=PLANE ( 'NONE',  #7178 ) ;
#3334=LINE ( 'NONE', #2221, #750 ) ;
#3338=VERTEX_POINT ( 'NONE', #772 ) ;
#3344=ORIENTED_EDGE ( 'NONE', *, *, #8568, .T. ) ;
#3356=AXIS2_PLACEMENT_3D ( 'NONE', #9673, #12880, #10843 ) ;
#3382=CARTESIAN_POINT ( 'NONE',  ( 52.44898870156725224, 66.83414752204051013, -1.000000000000000222 ) ) ;
#3388=CARTESIAN_POINT ( 'NONE',  ( 35.00000000000000000, 90.00000000000000000, 1.000000000000003109 ) ) ;
#3394=CARTESIAN_POINT ( 'NONE',  ( 35.00000000000000000, 90.00000000000000000, 4.000000000000000000 ) ) ;
#3403=ADVANCED_FACE ( 'NONE', ( #7841 ), #3070, .F. ) ;
#3411=ORIENTED_EDGE ( 'NONE', *, *, #7459, .T. ) ;
#3416=CARTESIAN_POINT ( 'NONE',  ( 53.69851220231782207, 63.41305505666788633, 1.000000000000003109 ) ) ;
#3427=AXIS2_PLACEMENT_3D ( 'NONE', #1857, #8851, #10876 ) ;
#3428=DIRECTION ( 'NONE',  ( 0.000000000000000000, 0.000000000000000000, -1.000000000000000000 ) ) ;
#3435=FACE_OUTER_BOUND ( 'NONE', #4962, .T. ) ;
#3444=CARTESIAN_POINT ( 'NONE',  ( 63.99885733073620742, 89.74256357754359215, -0.9999999999999970024 ) ) ;
#3447=DIRECTION ( 'NONE',  ( 1.000000000000000000, 0.000000000000000000, 0.000000000000000000 ) ) ;
#3452=CARTESIAN_POINT ( 'NONE',  ( 38.40477530926830951, 84.46307801270444315, 22.38477631085024555 ) ) ;
#3459=EDGE_CURVE ( 'NONE', #3150, #7702, #5281, .T. ) ;
#3474=CYLINDRICAL_SURFACE ( 'NONE', #8252, 30.00000000000000000 ) ;
#3482=EDGE_CURVE ( 'NONE', #11236, #955, #3334, .T. ) ;
#3484=PLANE ( 'NONE',  #11871 ) ;
#3489=VERTEX_POINT ( 'NONE', #11296 ) ;
#3502=DIRECTION ( 'NONE',  ( -0.5877852522924753575, 0.8090169943749458970, 0.000000000000000000 ) ) ;
#3503=DIRECTION ( 'NONE',  ( 1.000000000000000000, 2.135044278125301343E-15, 0.000000000000000000 ) ) ;
#3508=ADVANCED_FACE ( 'NONE', ( #9074 ), #229, .F. ) ;
#3510=DIRECTION ( 'NONE',  ( -0.000000000000000000, -0.000000000000000000, -1.000000000000000000 ) ) ;
#3512=CARTESIAN_POINT ( 'NONE',  ( 65.00000000000000000, 90.00000000000000000, -0.9999999999999970024 ) ) ;
#3516=LINE ( 'NONE', #9651, #7615 ) ;
#3543=ORIENTED_EDGE ( 'NONE', *, *, #2598, .F. ) ;
#3545=ORIENTED_EDGE ( 'NONE', *, *, #3949, .F. ) ;
#3548=VECTOR ( 'NONE', #10623, 1000.000000000000000 ) ;
#3554=EDGE_CURVE ( 'NONE', #5411, #10403, #11409, .T. ) ;
#3562=DIRECTION ( 'NONE',  ( -1.000000000000000000, 0.000000000000000000, 0.000000000000000000 ) ) ;
#3579=SURFACE_SIDE_STYLE ('',( #12537 ) ) ;
#3580=EDGE_CURVE ( 'NONE', #10434, #7702, #9464, .T. ) ;
#3583=CARTESIAN_POINT ( 'NONE',  ( 35.49992570027444572, 118.9956906159209069, 2.000000000000002220 ) ) ;
#3597=ADVANCED_FACE ( 'NONE', ( #4567 ), #7443, .T. ) ;
#3598=CARTESIAN_POINT ( 'NONE',  ( 35.00000000000000000, 90.00000000000000000, -3.000000000000000000 ) ) ;
#3605=ORIENTED_EDGE ( 'NONE', *, *, #7854, .F. ) ;
#3609=EDGE_CURVE ( 'NONE', #11688, #9045, #1172, .T. ) ;
#3615=AXIS2_PLACEMENT_3D ( 'NONE', #8531, #12518, #1655 ) ;
#3616=EDGE_CURVE ( 'NONE', #11952, #955, #1593, .T. ) ;
#3632=DIRECTION ( 'NONE',  ( 1.000000000000000000, 0.000000000000000000, 0.000000000000000000 ) ) ;
#3634=CARTESIAN_POINT ( 'NONE',  ( 34.49999999999995026, 119.0000000000000000, 4.000000000000000000 ) ) ;
#3635=VECTOR ( 'NONE', #2013, 1000.000000000000000 ) ;
#3665=CARTESIAN_POINT ( 'NONE',  ( 35.49999999999999289, 96.48074069840785683, -1.000000000000000000 ) ) ;
#3668=EDGE_LOOP ( 'NONE', ( #2888, #2572, #5845, #3411, #7997, #6613 ) ) ;
#3686=LINE ( 'NONE', #6676, #12740 ) ;
#3690=ORIENTED_EDGE ( 'NONE', *, *, #3026, .F. ) ;
#3698=DIRECTION ( 'NONE',  ( -1.000000000000000000, 0.000000000000000000, 0.000000000000000000 ) ) ;
#3699=FACE_OUTER_BOUND ( 'NONE', #3107, .T. ) ;
#3703=CARTESIAN_POINT ( 'NONE',  ( 35.00000000000000000, 90.00000000000000000, -3.000000000000000000 ) ) ;
#3708=VECTOR ( 'NONE', #5799, 1000.000000000000000 ) ;
#3709=CARTESIAN_POINT ( 'NONE',  ( 52.44898842787294768, 66.83414752756172561, 4.000000000000000000 ) ) ;
#3727=PLANE ( 'NONE',  #9381 ) ;
#3740=CARTESIAN_POINT ( 'NONE',  ( 41.00904217445251732, 92.47818727009297390, -0.9999999999999970024 ) ) ;
#3756=CARTESIAN_POINT ( 'NONE',  ( 35.00000000000000000, 90.00000000000000000, -1.000000000000000000 ) ) ;
#3757=EDGE_CURVE ( 'NONE', #11429, #10403, #5915, .T. ) ;
#3770=ORIENTED_EDGE ( 'NONE', *, *, #3301, .F. ) ;
#3775=CARTESIAN_POINT ( 'NONE',  ( -15.06519709809452756, 92.38262548349219117, 1.000000000000003109 ) ) ;
#3780=CARTESIAN_POINT ( 'NONE',  ( 65.00000000000000000, 117.5000000000001705, 1.000000000000003109 ) ) ;
#3781=EDGE_LOOP ( 'NONE', ( #11836, #8051, #348, #12465, #2414, #196, #9565, #9483 ) ) ;
#3789=DIRECTION ( 'NONE',  ( -0.8090169943749485615, 0.5877852522924716938, 0.000000000000000000 ) ) ;
#3798=VECTOR ( 'NONE', #12583, 999.9999999999998863 ) ;
#3801=ORIENTED_EDGE ( 'NONE', *, *, #2598, .T. ) ;
#3814=ADVANCED_FACE ( 'NONE', ( #9190 ), #12006, .T. ) ;
#3818=B_SPLINE_CURVE_WITH_KNOTS ( 'NONE', 3,
 ( #4354, #9189, #12463, #3382 ),
 .UNSPECIFIED., .F., .F.,
 ( 4, 4 ),
 ( 0.000000000000000000, 1.000000000000000000 ),
 .UNSPECIFIED. ) ;
#3821=CARTESIAN_POINT ( 'NONE',  ( 28.50000000000000355, 90.00000000000000000, -1.000000000000000888 ) ) ;
#3822=CARTESIAN_POINT ( 'NONE',  ( 35.75000000000000711, 93.41869858279433458, 22.38477631085024555 ) ) ;
#3830=EDGE_CURVE ( 'NONE', #7336, #11940, #3054, .T. ) ;
#3834=DIRECTION ( 'NONE',  ( -1.000000000000000000, 0.000000000000000000, 0.000000000000000000 ) ) ;
#3836=CARTESIAN_POINT ( 'NONE',  ( 7.266925296109192800, 98.48530998897412303, -1.000000000000000000 ) ) ;
#3856=AXIS2_PLACEMENT_3D ( 'NONE', #1869, #9972, #11743 ) ;
#3885=VECTOR ( 'NONE', #1664, 1000.000000000000000 ) ;
#3890=ADVANCED_FACE ( 'NONE', ( #6629 ), #12464, .F. ) ;
#3891=DIRECTION ( 'NONE',  ( -0.000000000000000000, -0.000000000000000000, -1.000000000000000000 ) ) ;
#3892=CARTESIAN_POINT ( 'NONE',  ( 18.35999867260799689, 66.24638416932324958, -1.000000000000000000 ) ) ;
#3906=AXIS2_PLACEMENT_3D ( 'NONE', #2525, #3510, #2394 ) ;
#3924=ORIENTED_EDGE ( 'NONE', *, *, #462, .T. ) ;
#3942=EDGE_LOOP ( 'NONE', ( #1502, #10128, #4621, #3058, #6530, #6932 ) ) ;
#3944=CARTESIAN_POINT ( 'NONE',  ( 35.00000000000000000, 90.00000000000000000, 4.000000000000000000 ) ) ;
#3949=EDGE_CURVE ( 'NONE', #4463, #4318, #12470, .T. ) ;
#3950=CIRCLE ( 'NONE', #1218, 29.99999999999999645 ) ;
#3967=CARTESIAN_POINT ( 'NONE',  ( 35.00000000000000000, 90.00000000000000000, 22.38477631085024555 ) ) ;
#3982=AXIS2_PLACEMENT_3D ( 'NONE', #1402, #12333, #10298 ) ;
#3994=AXIS2_PLACEMENT_3D ( 'NONE', #3703, #8665, #7617 ) ;
#3998=DIRECTION ( 'NONE',  ( -1.000000000000000000, 0.000000000000000000, 0.000000000000000000 ) ) ;
#4011=B_SPLINE_CURVE_WITH_KNOTS ( 'NONE', 3,
 ( #1477, #11486, #3583, #5662 ),
 .UNSPECIFIED., .F., .F.,
 ( 4, 4 ),
 ( 0.000000000000000000, 0.5999999999999994227 ),
 .UNSPECIFIED. ) ;
#4013=AXIS2_PLACEMENT_3D ( 'NONE', #1225, #5456, #12158 ) ;
#4019=VERTEX_POINT ( 'NONE', #7944 ) ;
#4025=VERTEX_POINT ( 'NONE', #10817 ) ;
#4029=DIRECTION ( 'NONE',  ( -1.000000000000000000, 0.000000000000000000, 0.000000000000000000 ) ) ;
#4037=CARTESIAN_POINT ( 'NONE',  ( 35.49999999999995026, 119.0000000000000000, -1.000000000000000000 ) ) ;
#4052=DIRECTION ( 'NONE',  ( -1.000000000000000000, 0.000000000000000000, 0.000000000000000000 ) ) ;
#4056=VERTEX_POINT ( 'NONE', #2189 ) ;
#4064=ORIENTED_EDGE ( 'NONE', *, *, #707, .F. ) ;
#4066=ORIENTED_EDGE ( 'NONE', *, *, #2241, .T. ) ;
#4067=EDGE_CURVE ( 'NONE', #1627, #4019, #10483, .T. ) ;
#4069=CIRCLE ( 'NONE', #3856, 29.99999999999999645 ) ;
#4071=MECHANICAL_DESIGN_GEOMETRIC_PRESENTATION_REPRESENTATION('',(#9491),#493);
#4076=VERTEX_POINT ( 'NONE', #2512 ) ;
#4081=EDGE_LOOP ( 'NONE', ( #3032, #2475, #758, #4775 ) ) ;
#4102=ORIENTED_EDGE ( 'NONE', *, *, #7335, .F. ) ;
#4104=VERTEX_POINT ( 'NONE', #12517 ) ;
#4116=CARTESIAN_POINT ( 'NONE',  ( 62.73514746974691292, 98.48596457872595522, 4.000000000000000000 ) ) ;
#4118=CYLINDRICAL_SURFACE ( 'NONE', #6528, 30.00000000000000000 ) ;
#4131=FACE_BOUND ( 'NONE', #5458, .T. ) ;
#4133=ORIENTED_EDGE ( 'NONE', *, *, #9196, .F. ) ;
#4137=CARTESIAN_POINT ( 'NONE',  ( 6.626776019045580668, 99.74475042915889844, 1.000000000000003109 ) ) ;
#4148=VERTEX_POINT ( 'NONE', #6360 ) ;
#4151=ORIENTED_EDGE ( 'NONE', *, *, #8018, .T. ) ;
#4154=EDGE_CURVE ( 'NONE', #6792, #8177, #10375, .T. ) ;
#4165=DIRECTION ( 'NONE',  ( -0.8090169943749457859, -0.5877852522924753575, 0.000000000000000000 ) ) ;
#4166=EDGE_LOOP ( 'NONE', ( #9813, #8577, #3011, #10516 ) ) ;
#4171=CIRCLE ( 'NONE', #12530, 28.99999999999999289 ) ;
#4191=ORIENTED_EDGE ( 'NONE', *, *, #8194, .F. ) ;
#4199=CYLINDRICAL_SURFACE ( 'NONE', #1280, 3.499999999999996003 ) ;
#4205=ORIENTED_EDGE ( 'NONE', *, *, #3609, .F. ) ;
#4210=VERTEX_POINT ( 'NONE', #851 ) ;
#4213=EDGE_CURVE ( 'NONE', #2081, #12892, #10865, .T. ) ;
#4214=CARTESIAN_POINT ( 'NONE',  ( 63.68224097532933570, 98.79369391286387270, 1.000000000000003109 ) ) ;
#4221=CYLINDRICAL_SURFACE ( 'NONE', #8527, 28.99999999999999289 ) ;
#4239=DIRECTION ( 'NONE',  ( 0.5877852522924753575, -0.8090169943749457859, 0.000000000000000000 ) ) ;
#4242=CARTESIAN_POINT ( 'NONE',  ( 34.50001850811341342, 118.9978265420697170, -1.000000000000000000 ) ) ;
#4252=EDGE_CURVE ( 'NONE', #1224, #4148, #970, .T. ) ;
#4261=FACE_BOUND ( 'NONE', #6455, .T. ) ;
#4262=LINE ( 'NONE', #9354, #6251 ) ;
#4264=FACE_OUTER_BOUND ( 'NONE', #12945, .T. ) ;
#4270=VERTEX_POINT ( 'NONE', #2899 ) ;
#4285=AXIS2_PLACEMENT_3D ( 'NONE', #5898, #4801, #12781 ) ;
#4291=LINE ( 'NONE', #1204, #1121 ) ;
#4315=LINE ( 'NONE', #9470, #11664 ) ;
#4316=EDGE_LOOP ( 'NONE', ( #8648, #4133, #7628, #10875 ) ) ;
#4318=VERTEX_POINT ( 'NONE', #10678 ) ;
#4329=DIRECTION ( 'NONE',  ( 0.000000000000000000, 0.000000000000000000, -1.000000000000000000 ) ) ;
#4348=VECTOR ( 'NONE', #10092, 1000.000000000000114 ) ;
#4354=CARTESIAN_POINT ( 'NONE',  ( 52.44898842787294768, 66.83414752756172561, 4.000000000000000000 ) ) ;
#4365=CARTESIAN_POINT ( 'NONE',  ( 17.55098605904792564, 66.83414348997642662, 1.000000000000003109 ) ) ;
#4367=ORIENTED_EDGE ( 'NONE', *, *, #12144, .F. ) ;
#4370=ORIENTED_EDGE ( 'NONE', *, *, #7869, .F. ) ;
#4376=CIRCLE ( 'NONE', #5207, 29.99999999999999645 ) ;
#4393=VECTOR ( 'NONE', #9992, 1000.000000000000000 ) ;
#4399=ORIENTED_EDGE ( 'NONE', *, *, #10311, .F. ) ;
#4400=DIRECTION ( 'NONE',  ( -0.9510565162951529761, -0.3090169943749492276, 0.000000000000000000 ) ) ;
#4405=DIRECTION ( 'NONE',  ( -0.000000000000000000, -0.000000000000000000, -1.000000000000000000 ) ) ;
#4418=AXIS2_PLACEMENT_3D ( 'NONE', #3944, #7926, #11913 ) ;
#4429=DIRECTION ( 'NONE',  ( -0.000000000000000000, -0.000000000000000000, -1.000000000000000000 ) ) ;
#4436=DIRECTION ( 'NONE',  ( 1.000000000000000000, 0.000000000000000000, 0.000000000000000000 ) ) ;
#4441=CARTESIAN_POINT ( 'NONE',  ( 35.00000000000000000, 90.00000000000000000, 4.000000000000000000 ) ) ;
#4445=CIRCLE ( 'NONE', #5279, 28.99999999999999289 ) ;
#4461=ORIENTED_EDGE ( 'NONE', *, *, #4715, .F. ) ;
#4462=DIRECTION ( 'NONE',  ( -0.5877852522924755796, -0.8090169943749457859, 0.000000000000000000 ) ) ;
#4463=VERTEX_POINT ( 'NONE', #6648 ) ;
#4474=CARTESIAN_POINT ( 'NONE',  ( 35.00000000000000000, 90.00000000000000000, 22.38477631085024555 ) ) ;
#4476=PLANE ( 'NONE',  #7292 ) ;
#4482=ORIENTED_EDGE ( 'NONE', *, *, #4582, .T. ) ;
#4502=ORIENTED_EDGE ( 'NONE', *, *, #10990, .T. ) ;
#4514=CARTESIAN_POINT ( 'NONE',  ( 6.626776019045581556, 99.74475042915889844, -0.9999999999999970024 ) ) ;
#4530=ORIENTED_EDGE ( 'NONE', *, *, #8611, .F. ) ;
#4533=ORIENTED_EDGE ( 'NONE', *, *, #707, .T. ) ;
#4542=LINE ( 'NONE', #10427, #5528 ) ;
#4557=EDGE_CURVE ( 'NONE', #8368, #4056, #7777, .T. ) ;
#4559=ADVANCED_FACE ( 'NONE', ( #4883 ), #8872, .F. ) ;
#4562=AXIS2_PLACEMENT_3D ( 'NONE', #3598, #4703, #7643 ) ;
#4567=FACE_OUTER_BOUND ( 'NONE', #3287, .T. ) ;
#4582=EDGE_CURVE ( 'NONE', #3017, #36, #2798, .T. ) ;
#4585=VECTOR ( 'NONE', #11137, 1000.000000000000000 ) ;
#4595=FACE_OUTER_BOUND ( 'NONE', #12141, .T. ) ;
#4607=DIRECTION ( 'NONE',  ( -1.000000000000000000, 0.000000000000000000, 0.000000000000000000 ) ) ;
#4611=CARTESIAN_POINT ( 'NONE',  ( 18.35873618070580093, 66.24461453698026503, -1.000000000000000000 ) ) ;
#4617=ORIENTED_EDGE ( 'NONE', *, *, #10184, .F. ) ;
#4621=ORIENTED_EDGE ( 'NONE', *, *, #1518, .F. ) ;
#4624=CARTESIAN_POINT ( 'NONE',  ( 35.75000000000000711, 93.50000000000000000, 4.000000000000000000 ) ) ;
#4626=ORIENTED_EDGE ( 'NONE', *, *, #10354, .T. ) ;
#4649=ORIENTED_EDGE ( 'NONE', *, *, #8701, .T. ) ;
#4665=CARTESIAN_POINT ( 'NONE',  ( 46.98957880828161393, 117.5000000000000711, 1.000000000000003553 ) ) ;
#4694=DIRECTION ( 'NONE',  ( -0.000000000000000000, -0.000000000000000000, -1.000000000000000000 ) ) ;
#4700=EDGE_CURVE ( 'NONE', #36, #5747, #1400, .T. ) ;
#4703=DIRECTION ( 'NONE',  ( 0.000000000000000000, 0.000000000000000000, -1.000000000000000000 ) ) ;
#4706=FACE_OUTER_BOUND ( 'NONE', #8283, .T. ) ;
#4715=EDGE_CURVE ( 'NONE', #7663, #1018, #5331, .T. ) ;
#4726=ORIENTED_EDGE ( 'NONE', *, *, #7635, .T. ) ;
#4736=CARTESIAN_POINT ( 'NONE',  ( 7.576448291486922670, 99.43666122937791840, 4.000000000000000000 ) ) ;
#4737=CARTESIAN_POINT ( 'NONE',  ( 18.35999869903453430, 66.24638416994363865, 4.000000000000000000 ) ) ;
#4743=VERTEX_POINT ( 'NONE', #12337 ) ;
#4768=DIRECTION ( 'NONE',  ( 0.000000000000000000, 0.000000000000000000, -1.000000000000000000 ) ) ;
#4775=ORIENTED_EDGE ( 'NONE', *, *, #8076, .F. ) ;
#4777=VECTOR ( 'NONE', #9984, 1000.000000000000000 ) ;
#4786=ORIENTED_EDGE ( 'NONE', *, *, #2930, .F. ) ;
#4790=DIRECTION ( 'NONE',  ( 0.5877852522924715828, 0.8090169943749485615, 0.000000000000000000 ) ) ;
#4801=DIRECTION ( 'NONE',  ( 0.000000000000000000, 0.000000000000000000, -1.000000000000000000 ) ) ;
#4804=CYLINDRICAL_SURFACE ( 'NONE', #1591, 6.499999999999999112 ) ;
#4823=ORIENTED_EDGE ( 'NONE', *, *, #440, .F. ) ;
#4824=DIRECTION ( 'NONE',  ( 0.000000000000000000, 0.000000000000000000, 1.000000000000000000 ) ) ;
#4831=PLANE ( 'NONE',  #11175 ) ;
#4834=CARTESIAN_POINT ( 'NONE',  ( 34.25000000000000000, 93.41869858279433458, 4.000000000000000000 ) ) ;
#4860=ORIENTED_EDGE ( 'NONE', *, *, #10676, .T. ) ;
#4862=CARTESIAN_POINT ( 'NONE',  ( 51.63999694657688622, 66.24635823768382181, 1.000000000000003109 ) ) ;
#4864=DIRECTION ( 'NONE',  ( -0.000000000000000000, -0.000000000000000000, -1.000000000000000000 ) ) ;
#4865=ORIENTED_EDGE ( 'NONE', *, *, #8970, .T. ) ;
#4871=VERTEX_POINT ( 'NONE', #9524 ) ;
#4883=FACE_OUTER_BOUND ( 'NONE', #3942, .T. ) ;
#4886=DIRECTION ( 'NONE',  ( 1.000000000000000000, 0.000000000000000000, 0.000000000000000000 ) ) ;
#4891=CARTESIAN_POINT ( 'NONE',  ( 34.49999999999995026, 119.0000000000000000, 0.6666666666666665186 ) ) ;
#4893=CIRCLE ( 'NONE', #2613, 30.00000000000000000 ) ;
#4897=CIRCLE ( 'NONE', #2187, 29.99999999999999645 ) ;
#4923=ORIENTED_EDGE ( 'NONE', *, *, #3091, .F. ) ;
#4925=DIRECTION ( 'NONE',  ( 0.000000000000000000, 0.000000000000000000, 1.000000000000000000 ) ) ;
#4927=ORIENTED_EDGE ( 'NONE', *, *, #6427, .T. ) ;
#4939=DIRECTION ( 'NONE',  ( 0.000000000000000000, -0.000000000000000000, -1.000000000000000000 ) ) ;
#4940=DIRECTION ( 'NONE',  ( -0.000000000000000000, 0.000000000000000000, 1.000000000000000000 ) ) ;
#4950=EDGE_CURVE ( 'NONE', #4056, #1497, #1620, .T. ) ;
#4962=EDGE_LOOP ( 'NONE', ( #3543, #11846, #614, #6505, #10600, #8324 ) ) ;
#4993=DIRECTION ( 'NONE',  ( -1.000000000000000000, 9.570888143320317860E-16, 0.000000000000000000 ) ) ;
#5016=ADVANCED_FACE ( 'NONE', ( #6 ), #805, .F. ) ;
#5019=CARTESIAN_POINT ( 'NONE',  ( 7.264852530253062213, 98.48596457872582732, 4.000000000000000000 ) ) ;
#5025=ORIENTED_EDGE ( 'NONE', *, *, #7115, .T. ) ;
#5027=AXIS2_PLACEMENT_3D ( 'NONE', #69, #10028, #7021 ) ;
#5038=ORIENTED_EDGE ( 'NONE', *, *, #6229, .F. ) ;
#5052=DIRECTION ( 'NONE',  ( 0.000000000000000000, 0.000000000000000000, 1.000000000000000000 ) ) ;
#5067=EDGE_CURVE ( 'NONE', #9866, #7702, #7048, .T. ) ;
#5069=VERTEX_POINT ( 'NONE', #5849 ) ;
#5080=CARTESIAN_POINT ( 'NONE',  ( 35.00000000000000000, 90.00000000000000000, 1.000000000000003109 ) ) ;
#5085=FACE_BOUND ( 'NONE', #4081, .T. ) ;
#5092=DIRECTION ( 'NONE',  ( -1.000000000000000000, 0.000000000000000000, 0.000000000000000000 ) ) ;
#5096=ORIENTED_EDGE ( 'NONE', *, *, #9242, .F. ) ;
#5099=ADVANCED_FACE ( 'NONE', ( #7153 ), #4221, .F. ) ;
#5125=( NAMED_UNIT ( * ) SI_UNIT ( $, .STERADIAN. ) SOLID_ANGLE_UNIT ( ) );
#5140=CARTESIAN_POINT ( 'NONE',  ( 17.54971918633085437, 66.83239978927272773, -1.000000000000000000 ) ) ;
#5142=CARTESIAN_POINT ( 'NONE',  ( 17.55231228847961944, 66.83584248194507893, 3.000000000000000888 ) ) ;
#5145=EDGE_CURVE ( 'NONE', #4056, #5747, #3243, .T. ) ;
#5146=CARTESIAN_POINT ( 'NONE',  ( 35.00000000000000000, 90.00000000000000000, 4.000000000000000000 ) ) ;
#5152=EDGE_LOOP ( 'NONE', ( #566, #3690, #5616, #9270, #2542, #10983 ) ) ;
#5168=LINE ( 'NONE', #2171, #9845 ) ;
#5170=AXIS2_PLACEMENT_3D ( 'NONE', #11414, #5457, #9452 ) ;
#5185=B_SPLINE_CURVE_WITH_KNOTS ( 'NONE', 3,
 ( #11797, #1855, #858, #4862 ),
 .UNSPECIFIED., .F., .F.,
 ( 4, 4 ),
 ( 0.000000000000000000, 0.5999999999999994227 ),
 .UNSPECIFIED. ) ;
#5203=CARTESIAN_POINT ( 'NONE',  ( 35.00000000000000000, 90.00000000000000000, -1.000000000000000888 ) ) ;
#5207=AXIS2_PLACEMENT_3D ( 'NONE', #5380, #7546, #4607 ) ;
#5208=DIRECTION ( 'NONE',  ( -0.5877852522924753575, 0.8090169943749458970, 0.000000000000000000 ) ) ;
#5216=DIRECTION ( 'NONE',  ( 0.9510565162951543083, -0.3090169943749451198, 0.000000000000000000 ) ) ;
#5220=ORIENTED_EDGE ( 'NONE', *, *, #7869, .T. ) ;
#5231=ORIENTED_EDGE ( 'NONE', *, *, #364, .F. ) ;
#5241=CARTESIAN_POINT ( 'NONE',  ( 35.49999999999995026, 118.9978446673979704, 1.000000000000003109 ) ) ;
#5261=AXIS2_PLACEMENT_3D ( 'NONE', #9808, #35, #4052 ) ;
#5273=CARTESIAN_POINT ( 'NONE',  ( 35.00000000000000000, 90.00000000000000000, 1.000000000000003109 ) ) ;
#5279=AXIS2_PLACEMENT_3D ( 'NONE', #10792, #1832, #7847 ) ;
#5281=LINE ( 'NONE', #7179, #7024 ) ;
#5320=LINE ( 'NONE', #267, #4585 ) ;
#5322=ADVANCED_FACE ( 'NONE', ( #2576 ), #6363, .T. ) ;
#5331=LINE ( 'NONE', #2274, #10386 ) ;
#5341=DIRECTION ( 'NONE',  ( -0.000000000000000000, -0.000000000000000000, -1.000000000000000000 ) ) ;
#5355=DIRECTION ( 'NONE',  ( 0.000000000000000000, 0.000000000000000000, -1.000000000000000000 ) ) ;
#5369=ORIENTED_EDGE ( 'NONE', *, *, #1250, .T. ) ;
#5375=DIRECTION ( 'NONE',  ( 0.000000000000000000, 0.000000000000000000, -1.000000000000000000 ) ) ;
#5380=CARTESIAN_POINT ( 'NONE',  ( 35.00000000000000000, 90.00000000000000000, 1.000000000000003553 ) ) ;
#5381=EDGE_CURVE ( 'NONE', #7791, #6015, #10211, .T. ) ;
#5388=VECTOR ( 'NONE', #6053, 1000.000000000000000 ) ;
#5396=CARTESIAN_POINT ( 'NONE',  ( 7.266925300896119211, 98.48530999652632545, 4.000000000000000000 ) ) ;
#5411=VERTEX_POINT ( 'NONE', #5241 ) ;
#5426=EDGE_LOOP ( 'NONE', ( #8513, #4502, #6856, #6611 ) ) ;
#5437=VECTOR ( 'NONE', #6837, 1000.000000000000000 ) ;
#5451=LINE ( 'NONE', #11607, #3885 ) ;
#5456=DIRECTION ( 'NONE',  ( -1.000000000000000000, 0.000000000000000000, -0.000000000000000000 ) ) ;
#5457=DIRECTION ( 'NONE',  ( 0.000000000000000000, 0.000000000000000000, 1.000000000000000000 ) ) ;
#5458=EDGE_LOOP ( 'NONE', ( #171, #6907, #8383, #7426, #1378, #8238 ) ) ;
#5462=DIRECTION ( 'NONE',  ( 1.000000000000000000, 0.000000000000000000, 0.000000000000000000 ) ) ;
#5470=EDGE_CURVE ( 'NONE', #7589, #7127, #11581, .T. ) ;
#5482=CARTESIAN_POINT ( 'NONE',  ( -15.06519709809452756, 92.38262548349219117, -0.9999999999999970024 ) ) ;
#5487=LINE ( 'NONE', #10532, #2215 ) ;
#5502=ORIENTED_EDGE ( 'NONE', *, *, #539, .T. ) ;
#5528=VECTOR ( 'NONE', #12656, 1000.000000000000000 ) ;
#5537=ORIENTED_EDGE ( 'NONE', *, *, #6307, .T. ) ;
#5542=EDGE_LOOP ( 'NONE', ( #9539, #4617, #11160, #2305 ) ) ;
#5548=EDGE_CURVE ( 'NONE', #1627, #1224, #1441, .T. ) ;
#5566=ORIENTED_EDGE ( 'NONE', *, *, #4067, .F. ) ;
#5574=CARTESIAN_POINT ( 'NONE',  ( 35.00000000000000000, 90.00000000000000000, 4.000000000000000000 ) ) ;
#5580=DIRECTION ( 'NONE',  ( 0.000000000000000000, 0.000000000000000000, -1.000000000000000000 ) ) ;
#5583=DIRECTION ( 'NONE',  ( -0.000000000000000000, -0.000000000000000000, -1.000000000000000000 ) ) ;
#5584=DIRECTION ( 'NONE',  ( 0.000000000000000000, 0.000000000000000000, -1.000000000000000000 ) ) ;
#5587=DIRECTION ( 'NONE',  ( -0.000000000000000000, -0.000000000000000000, -1.000000000000000000 ) ) ;
#5591=ORIENTED_EDGE ( 'NONE', *, *, #6607, .F. ) ;
#5595=AXIS2_PLACEMENT_3D ( 'NONE', #10555, #7479, #6620 ) ;
#5602=ADVANCED_FACE ( 'NONE', ( #7397 ), #3484, .F. ) ;
#5606=ORIENTED_EDGE ( 'NONE', *, *, #622, .T. ) ;
#5609=VERTEX_POINT ( 'NONE', #2694 ) ;
#5611=ORIENTED_EDGE ( 'NONE', *, *, #1120, .F. ) ;
#5616=ORIENTED_EDGE ( 'NONE', *, *, #8358, .F. ) ;
#5622=ORIENTED_EDGE ( 'NONE', *, *, #11633, .T. ) ;
#5646=DIRECTION ( 'NONE',  ( 0.000000000000000000, 0.000000000000000000, -1.000000000000000000 ) ) ;
#5662=CARTESIAN_POINT ( 'NONE',  ( 35.49999999999995026, 118.9978446673979704, 1.000000000000003109 ) ) ;
#5674=AXIS2_PLACEMENT_3D ( 'NONE', #9522, #3139, #3447 ) ;
#5676=B_SPLINE_CURVE_WITH_KNOTS ( 'NONE', 3,
 ( #11697, #5867, #4891, #2746 ),
 .UNSPECIFIED., .F., .F.,
 ( 4, 4 ),
 ( 0.000000000000000000, 1.000000000000000000 ),
 .UNSPECIFIED. ) ;
#5684=CARTESIAN_POINT ( 'NONE',  ( 51.63999694657688622, 66.24635823768382181, 1.000000000000003109 ) ) ;
#5697=CARTESIAN_POINT ( 'NONE',  ( 35.00000000000000000, 90.00000000000000000, 1.000000000000003109 ) ) ;
#5704=AXIS2_PLACEMENT_3D ( 'NONE', #8997, #4824, #4886 ) ;
#5716=CARTESIAN_POINT ( 'NONE',  ( 35.00000000000000000, 90.00000000000000000, -1.000000000000000888 ) ) ;
#5721=CARTESIAN_POINT ( 'NONE',  ( 35.00000000000000000, 90.00000000000000000, -1.000000000000000000 ) ) ;
#5736=DIRECTION ( 'NONE',  ( -1.000000000000000000, 0.000000000000000000, 0.000000000000000000 ) ) ;
#5743=CARTESIAN_POINT ( 'NONE',  ( 35.00000000000000000, 90.00000000000000000, -1.000000000000000000 ) ) ;
#5744=ORIENTED_EDGE ( 'NONE', *, *, #244, .F. ) ;
#5747=VERTEX_POINT ( 'NONE', #3740 ) ;
#5755=AXIS2_PLACEMENT_3D ( 'NONE', #6208, #239, #5092 ) ;
#5764=VECTOR ( 'NONE', #7563, 1000.000000000000000 ) ;
#5766=FACE_BOUND ( 'NONE', #11360, .T. ) ;
#5767=ORIENTED_EDGE ( 'NONE', *, *, #6976, .T. ) ;
#5773=AXIS2_PLACEMENT_3D ( 'NONE', #5080, #11491, #2413 ) ;
#5775=CARTESIAN_POINT ( 'NONE',  ( 6.000000000000008882, 90.00000000000000000, 4.000000000000000000 ) ) ;
#5777=DIRECTION ( 'NONE',  ( 0.000000000000000000, 0.000000000000000000, -1.000000000000000000 ) ) ;
#5799=DIRECTION ( 'NONE',  ( 1.914177628664063178E-15, -1.000000000000000000, 0.000000000000000000 ) ) ;
#5803=CARTESIAN_POINT ( 'NONE',  ( 13.22666678878058200, 110.6378768499380527, -3.000000000000000000 ) ) ;
#5805=DIRECTION ( 'NONE',  ( 0.000000000000000000, 0.000000000000000000, 1.000000000000000000 ) ) ;
#5806=FACE_OUTER_BOUND ( 'NONE', #11957, .T. ) ;
#5811=CARTESIAN_POINT ( 'NONE',  ( 28.50000000000000355, 90.00000000000000000, 4.000000000000000000 ) ) ;
#5821=EDGE_CURVE ( 'NONE', #3489, #587, #3950, .T. ) ;
#5840=CARTESIAN_POINT ( 'NONE',  ( 31.59522469073172601, 84.46307801270442894, -0.9999999999999970024 ) ) ;
#5844=DIRECTION ( 'NONE',  ( 1.000000000000000000, 0.000000000000000000, 0.000000000000000000 ) ) ;
#5845=ORIENTED_EDGE ( 'NONE', *, *, #349, .T. ) ;
#5848=ORIENTED_EDGE ( 'NONE', *, *, #8018, .F. ) ;
#5849=CARTESIAN_POINT ( 'NONE',  ( 62.73309762663101452, 98.48529854432332797, 1.000000000000003109 ) ) ;
#5852=FACE_OUTER_BOUND ( 'NONE', #5542, .T. ) ;
#5867=CARTESIAN_POINT ( 'NONE',  ( 34.49999999999995026, 119.0000000000000000, 2.333333333333333481 ) ) ;
#5877=CARTESIAN_POINT ( 'NONE',  ( 65.00000000000000000, 117.5000000000001705, 1.000000000000003109 ) ) ;
#5885=VERTEX_POINT ( 'NONE', #12161 ) ;
#5896=CARTESIAN_POINT ( 'NONE',  ( 35.75000000000000711, 92.49999999999998579, 4.000000000000000000 ) ) ;
#5898=CARTESIAN_POINT ( 'NONE',  ( 35.00000000000000000, 90.00000000000000000, 1.000000000000003553 ) ) ;
#5902=ORIENTED_EDGE ( 'NONE', *, *, #6427, .F. ) ;
#5913=LINE ( 'NONE', #3775, #6177 ) ;
#5914=CARTESIAN_POINT ( 'NONE',  ( 63.99885733073619321, 89.74256357754357794, 1.000000000000003109 ) ) ;
#5915=LINE ( 'NONE', #3780, #1600 ) ;
#5920=CARTESIAN_POINT ( 'NONE',  ( 38.50000000000000000, 90.00000000000000000, 4.000000000000000000 ) ) ;
#5938=DIRECTION ( 'NONE',  ( 1.000000000000000000, 0.000000000000000000, 0.000000000000000000 ) ) ;
#5942=AXIS2_PLACEMENT_3D ( 'NONE', #5697, #7851, #1899 ) ;
#5951=AXIS2_PLACEMENT_3D ( 'NONE', #2158, #12837, #3998 ) ;
#5958=CARTESIAN_POINT ( 'NONE',  ( 6.000000000000008882, 90.00000000000000000, -1.000000000000000000 ) ) ;
#5967=FACE_OUTER_BOUND ( 'NONE', #7059, .T. ) ;
#5978=EDGE_CURVE ( 'NONE', #9167, #4104, #1002, .T. ) ;
#5985=ORIENTED_EDGE ( 'NONE', *, *, #8530, .T. ) ;
#5995=LINE ( 'NONE', #2218, #4393 ) ;
#6014=CIRCLE ( 'NONE', #4562, 29.99999999999999645 ) ;
#6015=VERTEX_POINT ( 'NONE', #10391 ) ;
#6025=EDGE_CURVE ( 'NONE', #4270, #5411, #4315, .T. ) ;
#6027=DIRECTION ( 'NONE',  ( -1.000000000000000000, 0.000000000000000000, 0.000000000000000000 ) ) ;
#6029=EDGE_LOOP ( 'NONE', ( #4927, #12169, #6569, #7909 ) ) ;
#6030=CARTESIAN_POINT ( 'NONE',  ( 28.99095782554746847, 92.47818727009294548, 22.38477631085024555 ) ) ;
#6033=VECTOR ( 'NONE', #7801, 1000.000000000000000 ) ;
#6034=CARTESIAN_POINT ( 'NONE',  ( 35.49999999999995026, 119.0000000000000000, 4.000000000000000000 ) ) ;
#6041=VECTOR ( 'NONE', #10477, 1000.000000000000000 ) ;
#6044=DIRECTION ( 'NONE',  ( 0.000000000000000000, 0.000000000000000000, -1.000000000000000000 ) ) ;
#6048=ORIENTED_EDGE ( 'NONE', *, *, #8793, .T. ) ;
#6053=DIRECTION ( 'NONE',  ( -0.000000000000000000, -0.000000000000000000, -1.000000000000000000 ) ) ;
#6056=CARTESIAN_POINT ( 'NONE',  ( 18.35873618070580093, 66.24461453698026503, 4.000000000000000000 ) ) ;
#6069=DIRECTION ( 'NONE',  ( -1.000000000000000000, -5.551115123125781124E-15, 0.000000000000000000 ) ) ;
#6075=PLANE ( 'NONE',  #5755 ) ;
#6089=ORIENTED_EDGE ( 'NONE', *, *, #244, .T. ) ;
#6107=LINE ( 'NONE', #11213, #1338 ) ;
#6139=EDGE_LOOP ( 'NONE', ( #8446, #1686, #9060, #1035, #372, #11283 ) ) ;
#6147=CARTESIAN_POINT ( 'NONE',  ( 41.31805916882747454, 91.52713075379783447, 4.000000000000000000 ) ) ;
#6153=EDGE_LOOP ( 'NONE', ( #924, #3801, #7341, #5591 ) ) ;
#6158=CARTESIAN_POINT ( 'NONE',  ( 46.98957880828161393, 117.5000000000000711, -3.000000000000000000 ) ) ;
#6159=VERTEX_POINT ( 'NONE', #1065 ) ;
#6167=ORIENTED_EDGE ( 'NONE', *, *, #1120, .T. ) ;
#6177=VECTOR ( 'NONE', #9908, 1000.000000000000114 ) ;
#6208=CARTESIAN_POINT ( 'NONE',  ( 77.59086064835547347, 64.09101861717452664, 1.000000000000003109 ) ) ;
#6212=ADVANCED_FACE ( 'NONE', ( #6716 ), #631, .T. ) ;
#6216=ORIENTED_EDGE ( 'NONE', *, *, #1524, .T. ) ;
#6227=AXIS2_PLACEMENT_3D ( 'NONE', #3388, #219, #352 ) ;
#6229=EDGE_CURVE ( 'NONE', #8130, #10434, #6869, .T. ) ;
#6251=VECTOR ( 'NONE', #2304, 1000.000000000000000 ) ;
#6257=DIRECTION ( 'NONE',  ( -1.000000000000000000, 0.000000000000000000, 0.000000000000000000 ) ) ;
#6260=AXIS2_PLACEMENT_3D ( 'NONE', #3394, #5341, #6513 ) ;
#6272=VERTEX_POINT ( 'NONE', #6300 ) ;
#6279=VERTEX_POINT ( 'NONE', #11273 ) ;
#6300=CARTESIAN_POINT ( 'NONE',  ( 13.95244456248789788, 109.9499476216067819, 1.000000000000003109 ) ) ;
#6307=EDGE_CURVE ( 'NONE', #8177, #4318, #5320, .T. ) ;
#6310=ORIENTED_EDGE ( 'NONE', *, *, #2455, .F. ) ;
#6323=CARTESIAN_POINT ( 'NONE',  ( 35.75000000000000711, 92.49999999999998579, -4.802775637732004554 ) ) ;
#6336=VERTEX_POINT ( 'NONE', #9116 ) ;
#6342=EDGE_CURVE ( 'NONE', #10466, #8102, #9181, .T. ) ;
#6348=PRODUCT_DEFINITION_FORMATION_WITH_SPECIFIED_SOURCE ( 'ANY', '', #8352, .NOT_KNOWN. ) ;
#6355=PRODUCT_DEFINITION_SHAPE ( 'NONE', 'NONE',  #12256 ) ;
#6360=CARTESIAN_POINT ( 'NONE',  ( 43.71630314554308683, 62.34089554097972297, 1.000000000000003109 ) ) ;
#6363=CYLINDRICAL_SURFACE ( 'NONE', #5595, 6.499999999999999112 ) ;
#6369=PLANE ( 'NONE',  #10539 ) ;
#6380=LINE ( 'NONE', #1281, #7695 ) ;
#6384=ORIENTED_EDGE ( 'NONE', *, *, #10311, .T. ) ;
#6399=ORIENTED_EDGE ( 'NONE', *, *, #3616, .T. ) ;
#6412=ORIENTED_EDGE ( 'NONE', *, *, #1030, .T. ) ;
#6420=DIRECTION ( 'NONE',  ( -0.000000000000000000, -0.000000000000000000, -1.000000000000000000 ) ) ;
#6426=DIRECTION ( 'NONE',  ( 0.3090169943749451753, 0.9510565162951544194, -0.000000000000000000 ) ) ;
#6427=EDGE_CURVE ( 'NONE', #4076, #6279, #6556, .T. ) ;
#6441=( NAMED_UNIT ( * ) SI_UNIT ( $, .STERADIAN. ) SOLID_ANGLE_UNIT ( ) );
#6455=EDGE_LOOP ( 'NONE', ( #5848, #3295, #4191, #4649 ) ) ;
#6464=LINE ( 'NONE', #9547, #1573 ) ;
#6482=ORIENTED_EDGE ( 'NONE', *, *, #7115, .F. ) ;
#6483=LINE ( 'NONE', #7404, #6041 ) ;
#6496=CARTESIAN_POINT ( 'NONE',  ( 7.266925296109192800, 98.48530998897412303, -1.000000000000000000 ) ) ;
#6505=ORIENTED_EDGE ( 'NONE', *, *, #7629, .T. ) ;
#6513=DIRECTION ( 'NONE',  ( 1.000000000000000000, 0.000000000000000000, 0.000000000000000000 ) ) ;
#6528=AXIS2_PLACEMENT_3D ( 'NONE', #2820, #11771, #5938 ) ;
#6529=DIRECTION ( 'NONE',  ( 1.000000000000000000, 0.000000000000000000, 0.000000000000000000 ) ) ;
#6530=ORIENTED_EDGE ( 'NONE', *, *, #2837, .T. ) ;
#6534=ORIENTED_EDGE ( 'NONE', *, *, #7294, .T. ) ;
#6540=CARTESIAN_POINT ( 'NONE',  ( 35.75000000000000711, 93.50000000000000000, -3.000000000000000000 ) ) ;
#6550=ORIENTED_EDGE ( 'NONE', *, *, #2837, .F. ) ;
#6552=CLOSED_SHELL ( 'NONE', ( #11674, #8030, #11398, #8916, #12572, #1112, #4559, #5099, #12746, #9252, #11872, #5602, #3890, #3403, #5016, #9315, #2664, #8843, #1395, #6797, #12499, #2966, #335, #3814, #221, #7883, #8738, #900, #607, #6212, #12571, #9144, #9590, #3597, #11005, #260, #12092, #8433, #2323, #5322, #10347, #9826, #7155, #7820, #11907, #579, #3508 ) ) ;
#6556=LINE ( 'NONE', #532, #2290 ) ;
#6564=CARTESIAN_POINT ( 'NONE',  ( 38.50000000000000000, 90.00000000000000000, 22.38477631085024555 ) ) ;
#6569=ORIENTED_EDGE ( 'NONE', *, *, #6342, .F. ) ;
#6573=LINE ( 'NONE', #4624, #3225 ) ;
#6586=CARTESIAN_POINT ( 'NONE',  ( 35.00000000000000000, 90.00000000000000000, -1.000000000000000888 ) ) ;
#6599=CIRCLE ( 'NONE', #11617, 6.499999999999999112 ) ;
#6607=EDGE_CURVE ( 'NONE', #10599, #6015, #314, .T. ) ;
#6609=VECTOR ( 'NONE', #3428, 1000.000000000000000 ) ;
#6611=ORIENTED_EDGE ( 'NONE', *, *, #9626, .F. ) ;
#6613=ORIENTED_EDGE ( 'NONE', *, *, #12600, .F. ) ;
#6620=DIRECTION ( 'NONE',  ( -1.000000000000000000, 0.000000000000000000, 0.000000000000000000 ) ) ;
#6629=FACE_OUTER_BOUND ( 'NONE', #3781, .T. ) ;
#6632=EDGE_CURVE ( 'NONE', #7517, #1497, #4262, .T. ) ;
#6642=VECTOR ( 'NONE', #3061, 1000.000000000000000 ) ;
#6645=CYLINDRICAL_SURFACE ( 'NONE', #11912, 6.499999999999999112 ) ;
#6647=ORIENTED_EDGE ( 'NONE', *, *, #6652, .F. ) ;
#6648=CARTESIAN_POINT ( 'NONE',  ( 38.40477530926831662, 84.46307801270444315, 4.000000000000000000 ) ) ;
#6652=EDGE_CURVE ( 'NONE', #619, #8267, #11533, .T. ) ;
#6657=ORIENTED_EDGE ( 'NONE', *, *, #5145, .T. ) ;
#6662=AXIS2_PLACEMENT_3D ( 'NONE', #6948, #2844, #6027 ) ;
#6666=EDGE_CURVE ( 'NONE', #12180, #1278, #1523, .T. ) ;
#6674=CARTESIAN_POINT ( 'NONE',  ( 16.96438320935645905, 66.02675393316422969, -3.000000000000000000 ) ) ;
#6676=CARTESIAN_POINT ( 'NONE',  ( 62.73514746974691292, 98.48596457872595522, -1.000000000000000000 ) ) ;
#6689=VECTOR ( 'NONE', #8405, 1000.000000000000000 ) ;
#6698=CIRCLE ( 'NONE', #10248, 3.499999999999996003 ) ;
#6702=CARTESIAN_POINT ( 'NONE',  ( 35.75000000000000711, 93.41869858279433458, -3.000000000000000000 ) ) ;
#6705=EDGE_CURVE ( 'NONE', #11236, #330, #4376, .T. ) ;
#6709=CARTESIAN_POINT ( 'NONE',  ( 35.00000000000000000, 90.00000000000000000, 4.000000000000000000 ) ) ;
#6716=FACE_OUTER_BOUND ( 'NONE', #1535, .T. ) ;
#6721=DIRECTION ( 'NONE',  ( 1.000000000000000000, 1.914177628664063178E-15, -0.000000000000000000 ) ) ;
#6722=EDGE_LOOP ( 'NONE', ( #3545, #903, #3000, #8917 ) ) ;
#6733=AXIS2_PLACEMENT_3D ( 'NONE', #5877, #10852, #6069 ) ;
#6736=EDGE_CURVE ( 'NONE', #8306, #8496, #12385, .T. ) ;
#6754=LINE ( 'NONE', #12842, #9912 ) ;
#6767=( NAMED_UNIT ( * ) PLANE_ANGLE_UNIT ( ) SI_UNIT ( $, .RADIAN. ) );
#6772=DIRECTION ( 'NONE',  ( -1.000000000000000000, 0.000000000000000000, -0.000000000000000000 ) ) ;
#6778=CIRCLE ( 'NONE', #8674, 6.499999999999999112 ) ;
#6787=ORIENTED_EDGE ( 'NONE', *, *, #10990, .F. ) ;
#6789=DIRECTION ( 'NONE',  ( 0.9510565162951543083, -0.3090169943749451198, 0.000000000000000000 ) ) ;
#6792=VERTEX_POINT ( 'NONE', #399 ) ;
#6797=ADVANCED_FACE ( 'NONE', ( #3435 ), #7416, .T. ) ;
#6808=ORIENTED_EDGE ( 'NONE', *, *, #7459, .F. ) ;
#6832=DIRECTION ( 'NONE',  ( 0.000000000000000000, 0.000000000000000000, -1.000000000000000000 ) ) ;
#6837=DIRECTION ( 'NONE',  ( -0.5877852522924753575, 0.8090169943749458970, 0.000000000000000000 ) ) ;
#6856=ORIENTED_EDGE ( 'NONE', *, *, #7250, .T. ) ;
#6857=DIRECTION ( 'NONE',  ( -1.000000000000000000, 0.000000000000000000, -0.000000000000000000 ) ) ;
#6869=CIRCLE ( 'NONE', #7288, 6.499999999999999112 ) ;
#6874=CARTESIAN_POINT ( 'NONE',  ( 62.73102604205943322, 98.48470356904833523, 3.000000000000000888 ) ) ;
#6877=AXIS2_PLACEMENT_3D ( 'NONE', #12444, #4462, #1647 ) ;
#6879=EDGE_CURVE ( 'NONE', #1672, #8022, #4171, .T. ) ;
#6884=CARTESIAN_POINT ( 'NONE',  ( 35.00000000000000000, 90.00000000000000000, -3.000000000000000000 ) ) ;
#6886=VERTEX_POINT ( 'NONE', #5958 ) ;
#6901=CIRCLE ( 'NONE', #1896, 30.00000000000000000 ) ;
#6902=CARTESIAN_POINT ( 'NONE',  ( 34.49999999999998579, 96.48074069840785683, -0.9999999999999970024 ) ) ;
#6907=ORIENTED_EDGE ( 'NONE', *, *, #4213, .F. ) ;
#6920=CARTESIAN_POINT ( 'NONE',  ( 35.00000000000000000, 90.00000000000000000, -1.000000000000000000 ) ) ;
#6926=FACE_OUTER_BOUND ( 'NONE', #9289, .T. ) ;
#6932=ORIENTED_EDGE ( 'NONE', *, *, #11469, .T. ) ;
#6937=ORIENTED_EDGE ( 'NONE', *, *, #3301, .T. ) ;
#6948=CARTESIAN_POINT ( 'NONE',  ( 35.00000000000000000, 90.00000000000000000, 1.000000000000003553 ) ) ;
#6951=AXIS2_PLACEMENT_3D ( 'NONE', #9469, #11430, #10707 ) ;
#6974=CARTESIAN_POINT ( 'NONE',  ( 34.25000000000000000, 92.49999999999998579, -4.802775637732004554 ) ) ;
#6975=CARTESIAN_POINT ( 'NONE',  ( 17.26299177799148055, 43.12143982588584379, 1.000000000000003109 ) ) ;
#6976=EDGE_CURVE ( 'NONE', #9073, #10434, #11255, .T. ) ;
#6979=AXIS2_PLACEMENT_3D ( 'NONE', #12001, #7753, #1805 ) ;
#6985=ORIENTED_EDGE ( 'NONE', *, *, #1995, .F. ) ;
#6988=FACE_BOUND ( 'NONE', #9654, .T. ) ;
#7012=AXIS2_PLACEMENT_3D ( 'NONE', #940, #7755, #12003 ) ;
#7016=LINE ( 'NONE', #3822, #8768 ) ;
#7019=FACE_OUTER_BOUND ( 'NONE', #7214, .T. ) ;
#7021=DIRECTION ( 'NONE',  ( 0.8090169943749476733, 0.5877852522924726930, 0.000000000000000000 ) ) ;
#7023=ORIENTED_EDGE ( 'NONE', *, *, #663, .F. ) ;
#7024=VECTOR ( 'NONE', #5216, 1000.000000000000000 ) ;
#7036=CARTESIAN_POINT ( 'NONE',  ( 15.49247080330699866, 64.00084030896054799, 1.000000000000003109 ) ) ;
#7042=LINE ( 'NONE', #11023, #5388 ) ;
#7048=CIRCLE ( 'NONE', #3092, 6.499999999999999112 ) ;
#7058=VECTOR ( 'NONE', #2369, 1000.000000000000227 ) ;
#7059=EDGE_LOOP ( 'NONE', ( #11310, #12843, #4923, #11651 ) ) ;
#7060=CARTESIAN_POINT ( 'NONE',  ( 35.00000000000000000, 90.00000000000000000, -1.000000000000000888 ) ) ;
#7074=SHAPE_REPRESENTATION_RELATIONSHIP ( 'NONE' , 'NONE' ,  #7342, #9016 ) ;
#7115=EDGE_CURVE ( 'NONE', #587, #3489, #6014, .T. ) ;
#7118=DIRECTION ( 'NONE',  ( -0.9510565162951529761, -0.3090169943749492276, 0.000000000000000000 ) ) ;
#7127=VERTEX_POINT ( 'NONE', #2743 ) ;
#7131=FACE_BOUND ( 'NONE', #2985, .T. ) ;
#7133=ORIENTED_EDGE ( 'NONE', *, *, #6879, .F. ) ;
#7144=DIRECTION ( 'NONE',  ( -0.000000000000000000, -0.000000000000000000, 1.000000000000000000 ) ) ;
#7153=FACE_OUTER_BOUND ( 'NONE', #6139, .T. ) ;
#7155=ADVANCED_FACE ( 'NONE', ( #567 ), #12307, .T. ) ;
#7178=AXIS2_PLACEMENT_3D ( 'NONE', #7368, #10379, #155 ) ;
#7179=CARTESIAN_POINT ( 'NONE',  ( 7.264852530253062213, 98.48596457872582732, 4.000000000000000000 ) ) ;
#7214=EDGE_LOOP ( 'NONE', ( #7520, #4860, #2540, #8204 ) ) ;
#7218=DIRECTION ( 'NONE',  ( 1.000000000000000000, 0.000000000000000000, 0.000000000000000000 ) ) ;
#7248=DIRECTION ( 'NONE',  ( 0.000000000000000000, 1.000000000000000000, -0.000000000000000000 ) ) ;
#7250=EDGE_CURVE ( 'NONE', #9471, #11248, #2012, .T. ) ;
#7260=PRODUCT_CONTEXT ( 'NONE', #1241, 'mechanical' ) ;
#7268=VECTOR ( 'NONE', #2245, 1000.000000000000000 ) ;
#7288=AXIS2_PLACEMENT_3D ( 'NONE', #6586, #10589, #5736 ) ;
#7292=AXIS2_PLACEMENT_3D ( 'NONE', #1597, #5584, #2456 ) ;
#7294=EDGE_CURVE ( 'NONE', #3489, #11952, #8999, .T. ) ;
#7302=VECTOR ( 'NONE', #5646, 1000.000000000000000 ) ;
#7305=DIRECTION ( 'NONE',  ( 0.000000000000000000, -0.000000000000000000, -1.000000000000000000 ) ) ;
#7310=VERTEX_POINT ( 'NONE', #2871 ) ;
#7330=CARTESIAN_POINT ( 'NONE',  ( 35.00000000000000000, 90.00000000000000000, 22.38477631085024555 ) ) ;
#7335=EDGE_CURVE ( 'NONE', #5885, #9045, #8812, .T. ) ;
#7336=VERTEX_POINT ( 'NONE', #8875 ) ;
#7341=ORIENTED_EDGE ( 'NONE', *, *, #10006, .T. ) ;
#7342=SHAPE_REPRESENTATION ( 'conveyor wheel', ( #5704 ), #2789 ) ;
#7347=EDGE_CURVE ( 'NONE', #6159, #7310, #7042, .T. ) ;
#7368=CARTESIAN_POINT ( 'NONE',  ( 20.20191803945384379, 39.07635485401110742, 1.000000000000003109 ) ) ;
#7394=EDGE_LOOP ( 'NONE', ( #6089, #2288, #7133, #10156, #4726, #1176 ) ) ;
#7397=FACE_OUTER_BOUND ( 'NONE', #1417, .T. ) ;
#7404=CARTESIAN_POINT ( 'NONE',  ( 34.25000000000000000, 93.50000000000000000, 4.000000000000000000 ) ) ;
#7408=CIRCLE ( 'NONE', #10541, 28.99999999999999289 ) ;
#7411=EDGE_CURVE ( 'NONE', #4019, #6792, #6380, .T. ) ;
#7416=PLANE ( 'NONE',  #12946 ) ;
#7426=ORIENTED_EDGE ( 'NONE', *, *, #11796, .F. ) ;
#7428=CIRCLE ( 'NONE', #12445, 30.00000000000000000 ) ;
#7443=PLANE ( 'NONE',  #7655 ) ;
#7459=EDGE_CURVE ( 'NONE', #11940, #6159, #8536, .T. ) ;
#7464=DIRECTION ( 'NONE',  ( -1.000000000000000000, 0.000000000000000000, -0.000000000000000000 ) ) ;
#7479=DIRECTION ( 'NONE',  ( -0.000000000000000000, -0.000000000000000000, -1.000000000000000000 ) ) ;
#7495=ORIENTED_EDGE ( 'NONE', *, *, #913, .F. ) ;
#7498=DIRECTION ( 'NONE',  ( 0.000000000000000000, 0.000000000000000000, 1.000000000000000000 ) ) ;
#7504=LINE ( 'NONE', #10446, #2519 ) ;
#7517=VERTEX_POINT ( 'NONE', #8290 ) ;
#7520=ORIENTED_EDGE ( 'NONE', *, *, #2366, .F. ) ;
#7529=VERTEX_POINT ( 'NONE', #12278 ) ;
#7540=CYLINDRICAL_SURFACE ( 'NONE', #2753, 6.499999999999999112 ) ;
#7542=PLANE ( 'NONE',  #871 ) ;
#7546=DIRECTION ( 'NONE',  ( -0.000000000000000000, 0.000000000000000000, -1.000000000000000000 ) ) ;
#7549=DIRECTION ( 'NONE',  ( 0.5877852522924715828, 0.8090169943749485615, 0.000000000000000000 ) ) ;
#7554=DIRECTION ( 'NONE',  ( 0.000000000000000000, 0.000000000000000000, -1.000000000000000000 ) ) ;
#7560=SURFACE_STYLE_USAGE ( .BOTH. , #3579 ) ;
#7563=DIRECTION ( 'NONE',  ( -0.000000000000000000, -0.000000000000000000, -1.000000000000000000 ) ) ;
#7565=ORIENTED_EDGE ( 'NONE', *, *, #4715, .T. ) ;
#7570=DIRECTION ( 'NONE',  ( 0.000000000000000000, -0.000000000000000000, 1.000000000000000000 ) ) ;
#7574=ORIENTED_EDGE ( 'NONE', *, *, #8672, .T. ) ;
#7578=DIRECTION ( 'NONE',  ( -1.000000000000000000, 0.000000000000000000, 0.000000000000000000 ) ) ;
#7586=ORIENTED_EDGE ( 'NONE', *, *, #2455, .T. ) ;
#7589=VERTEX_POINT ( 'NONE', #6702 ) ;
#7590=EDGE_CURVE ( 'NONE', #6792, #4463, #8416, .T. ) ;
#7604=FACE_OUTER_BOUND ( 'NONE', #8887, .T. ) ;
#7615=VECTOR ( 'NONE', #679, 1000.000000000000114 ) ;
#7617=DIRECTION ( 'NONE',  ( -1.000000000000000000, 0.000000000000000000, 0.000000000000000000 ) ) ;
#7626=DIRECTION ( 'NONE',  ( 0.000000000000000000, 0.000000000000000000, 1.000000000000000000 ) ) ;
#7628=ORIENTED_EDGE ( 'NONE', *, *, #8358, .T. ) ;
#7629=EDGE_CURVE ( 'NONE', #12180, #12399, #3516, .T. ) ;
#7635=EDGE_CURVE ( 'NONE', #7791, #4025, #7408, .T. ) ;
#7643=DIRECTION ( 'NONE',  ( -1.000000000000000000, 0.000000000000000000, 0.000000000000000000 ) ) ;
#7649=LINE ( 'NONE', #2877, #11901 ) ;
#7652=CIRCLE ( 'NONE', #12246, 30.00000000000000000 ) ;
#7655=AXIS2_PLACEMENT_3D ( 'NONE', #425, #8682, #1549 ) ;
#7663=VERTEX_POINT ( 'NONE', #3709 ) ;
#7679=CARTESIAN_POINT ( 'NONE',  ( 63.68224097532933570, 98.79369391286385849, -0.9999999999999970024 ) ) ;
#7693=CARTESIAN_POINT ( 'NONE',  ( 12.55092940903992194, 109.9007343985615393, -0.9999999999999970024 ) ) ;
#7695=VECTOR ( 'NONE', #5208, 1000.000000000000000 ) ;
#7702=VERTEX_POINT ( 'NONE', #1998 ) ;
#7709=ORIENTED_EDGE ( 'NONE', *, *, #9615, .T. ) ;
#7733=CARTESIAN_POINT ( 'NONE',  ( 35.00000000000000000, 90.00000000000000000, 22.38477631085024555 ) ) ;
#7735=FACE_OUTER_BOUND ( 'NONE', #6029, .T. ) ;
#7738=DIRECTION ( 'NONE',  ( -1.000000000000000000, 0.000000000000000000, 0.000000000000000000 ) ) ;
#7741=AXIS2_PLACEMENT_3D ( 'NONE', #1203, #9379, #2328 ) ;
#7749=CIRCLE ( 'NONE', #11291, 28.99999999999999289 ) ;
#7750=DIRECTION ( 'NONE',  ( -0.000000000000000000, -0.000000000000000000, -1.000000000000000000 ) ) ;
#7751=ORIENTED_EDGE ( 'NONE', *, *, #5381, .F. ) ;
#7753=DIRECTION ( 'NONE',  ( 0.000000000000000000, 0.000000000000000000, 1.000000000000000000 ) ) ;
#7755=DIRECTION ( 'NONE',  ( 0.000000000000000000, 0.000000000000000000, -1.000000000000000000 ) ) ;
#7768=DIRECTION ( 'NONE',  ( -0.5877852522924715828, -0.8090169943749484505, 0.000000000000000000 ) ) ;
#7777=B_SPLINE_CURVE_WITH_KNOTS ( 'NONE', 3,
 ( #12009, #10044, #12741, #2928 ),
 .UNSPECIFIED., .F., .F.,
 ( 4, 4 ),
 ( 0.000000000000000000, 1.000000000000000000 ),
 .UNSPECIFIED. ) ;
#7785=DIRECTION ( 'NONE',  ( 0.000000000000000000, 0.000000000000000000, -1.000000000000000000 ) ) ;
#7791=VERTEX_POINT ( 'NONE', #1868 ) ;
#7794=EDGE_CURVE ( 'NONE', #12180, #8074, #12638, .T. ) ;
#7797=AXIS2_PLACEMENT_3D ( 'NONE', #9154, #3087, #1174 ) ;
#7801=DIRECTION ( 'NONE',  ( -0.000000000000000000, -0.000000000000000000, 1.000000000000000000 ) ) ;
#7817=DIRECTION ( 'NONE',  ( -1.000000000000000000, 0.000000000000000000, -0.000000000000000000 ) ) ;
#7820=ADVANCED_FACE ( 'NONE', ( #5852 ), #3047, .F. ) ;
#7821=DIRECTION ( 'NONE',  ( -1.000000000000000000, 0.000000000000000000, 0.000000000000000000 ) ) ;
#7838=FACE_OUTER_BOUND ( 'NONE', #8247, .T. ) ;
#7841=FACE_OUTER_BOUND ( 'NONE', #10003, .T. ) ;
#7847=DIRECTION ( 'NONE',  ( -1.000000000000000000, 0.000000000000000000, 0.000000000000000000 ) ) ;
#7849=ORIENTED_EDGE ( 'NONE', *, *, #5067, .T. ) ;
#7850=MANIFOLD_SOLID_BREP ( 'Extrude-Thin4', #6552 ) ;
#7851=DIRECTION ( 'NONE',  ( -0.000000000000000000, 0.000000000000000000, -1.000000000000000000 ) ) ;
#7854=EDGE_CURVE ( 'NONE', #4270, #11429, #4897, .T. ) ;
#7869=EDGE_CURVE ( 'NONE', #5747, #7529, #9317, .T. ) ;
#7870=DIRECTION ( 'NONE',  ( 0.000000000000000000, 0.000000000000000000, 1.000000000000000000 ) ) ;
#7883=ADVANCED_FACE ( 'NONE', ( #12196 ), #8080, .T. ) ;
#7891=ORIENTED_EDGE ( 'NONE', *, *, #6705, .F. ) ;
#7898=DIRECTION ( 'NONE',  ( -0.3090169943749500048, 0.9510565162951528650, 0.000000000000000000 ) ) ;
#7909=ORIENTED_EDGE ( 'NONE', *, *, #11341, .F. ) ;
#7913=CARTESIAN_POINT ( 'NONE',  ( 35.75000000000000711, 92.49999999999998579, -3.000000000000000000 ) ) ;
#7916=VERTEX_POINT ( 'NONE', #1202 ) ;
#7926=DIRECTION ( 'NONE',  ( -0.000000000000000000, -0.000000000000000000, -1.000000000000000000 ) ) ;
#7927=DIRECTION ( 'NONE',  ( -1.000000000000000000, 0.000000000000000000, 0.000000000000000000 ) ) ;
#7931=VECTOR ( 'NONE', #465, 1000.000000000000000 ) ;
#7940=DIRECTION ( 'NONE',  ( 0.000000000000000000, 0.000000000000000000, 1.000000000000000000 ) ) ;
#7944=CARTESIAN_POINT ( 'NONE',  ( 52.22659979626835991, 65.43896868087158225, -0.9999999999999970024 ) ) ;
#7947=DIRECTION ( 'NONE',  ( 0.000000000000000000, 0.000000000000000000, -1.000000000000000000 ) ) ;
#7949=EDGE_CURVE ( 'NONE', #11775, #4871, #4542, .T. ) ;
#7957=ORIENTED_EDGE ( 'NONE', *, *, #1979, .T. ) ;
#7964=CARTESIAN_POINT ( 'NONE',  ( 35.00000000000000000, 90.00000000000000000, 4.000000000000000000 ) ) ;
#7968=DIRECTION ( 'NONE',  ( -0.000000000000000000, -0.000000000000000000, -1.000000000000000000 ) ) ;
#7969=ORIENTED_EDGE ( 'NONE', *, *, #9052, .T. ) ;
#7992=AXIS2_PLACEMENT_3D ( 'NONE', #2575, #1783, #3562 ) ;
#7997=ORIENTED_EDGE ( 'NONE', *, *, #7347, .T. ) ;
#8000=CYLINDRICAL_SURFACE ( 'NONE', #10854, 28.99999999999999289 ) ;
#8005=ORIENTED_EDGE ( 'NONE', *, *, #7250, .F. ) ;
#8009=ORIENTED_EDGE ( 'NONE', *, *, #8568, .F. ) ;
#8018=EDGE_CURVE ( 'NONE', #5609, #7529, #6778, .T. ) ;
#8022=VERTEX_POINT ( 'NONE', #9443 ) ;
#8030=ADVANCED_FACE ( 'NONE', ( #467 ), #2650, .F. ) ;
#8037=AXIS2_PLACEMENT_3D ( 'NONE', #8735, #4939, #4029 ) ;
#8040=ORIENTED_EDGE ( 'NONE', *, *, #4700, .F. ) ;
#8047=AXIS2_PLACEMENT_3D ( 'NONE', #9829, #4925, #10810 ) ;
#8051=ORIENTED_EDGE ( 'NONE', *, *, #1839, .T. ) ;
#8054=AXIS2_PLACEMENT_3D ( 'NONE', #5019, #889, #3065 ) ;
#8057=VECTOR ( 'NONE', #7785, 1000.000000000000000 ) ;
#8074=VERTEX_POINT ( 'NONE', #12523 ) ;
#8076=EDGE_CURVE ( 'NONE', #454, #1278, #2823, .T. ) ;
#8080=PLANE ( 'NONE',  #2411 ) ;
#8083=AXIS2_PLACEMENT_3D ( 'NONE', #1388, #5375, #9371 ) ;
#8087=VERTEX_POINT ( 'NONE', #5896 ) ;
#8092=DIRECTION ( 'NONE',  ( 0.5877852522924715828, 0.8090169943749485615, 0.000000000000000000 ) ) ;
#8094=ORIENTED_EDGE ( 'NONE', *, *, #440, .T. ) ;
#8102=VERTEX_POINT ( 'NONE', #3444 ) ;
#8104=FACE_OUTER_BOUND ( 'NONE', #5426, .T. ) ;
#8118=FACE_BOUND ( 'NONE', #518, .T. ) ;
#8121=AXIS2_PLACEMENT_3D ( 'NONE', #4441, #8370, #9343 ) ;
#8130=VERTEX_POINT ( 'NONE', #3821 ) ;
#8137=CIRCLE ( 'NONE', #6662, 29.99999999999999645 ) ;
#8148=CARTESIAN_POINT ( 'NONE',  ( 35.49999999999999289, 96.48074069840785683, 22.38477631085024555 ) ) ;
#8149=DIRECTION ( 'NONE',  ( 1.914177628664063178E-15, -1.000000000000000000, 0.000000000000000000 ) ) ;
#8150=DIRECTION ( 'NONE',  ( -0.000000000000000000, -0.000000000000000000, -1.000000000000000000 ) ) ;
#8177=VERTEX_POINT ( 'NONE', #5840 ) ;
#8194=EDGE_CURVE ( 'NONE', #8368, #1906, #11164, .T. ) ;
#8202=CARTESIAN_POINT ( 'NONE',  ( 35.00000000000000000, 90.00000000000000000, 4.000000000000000000 ) ) ;
#8204=ORIENTED_EDGE ( 'NONE', *, *, #10513, .F. ) ;
#8226=DIRECTION ( 'NONE',  ( 0.000000000000000000, 0.000000000000000000, 1.000000000000000000 ) ) ;
#8238=ORIENTED_EDGE ( 'NONE', *, *, #5067, .F. ) ;
#8247=EDGE_LOOP ( 'NONE', ( #5767, #784, #2007, #5606 ) ) ;
#8250=ORIENTED_EDGE ( 'NONE', *, *, #9626, .T. ) ;
#8252=AXIS2_PLACEMENT_3D ( 'NONE', #8438, #7144, #3100 ) ;
#8253=AXIS2_PLACEMENT_3D ( 'NONE', #4474, #5583, #3698 ) ;
#8264=ORIENTED_EDGE ( 'NONE', *, *, #5821, .F. ) ;
#8267=VERTEX_POINT ( 'NONE', #10412 ) ;
#8274=VECTOR ( 'NONE', #9527, 1000.000000000000000 ) ;
#8283=EDGE_LOOP ( 'NONE', ( #7709, #10392, #6647, #12364, #4786, #11169, #6399 ) ) ;
#8289=VECTOR ( 'NONE', #9056, 1000.000000000000114 ) ;
#8290=CARTESIAN_POINT ( 'NONE',  ( 46.98957880828161393, 117.5000000000000711, -0.9999999999999970024 ) ) ;
#8292=DIRECTION ( 'NONE',  ( -1.000000000000000000, 0.000000000000000000, 0.000000000000000000 ) ) ;
#8293=UNCERTAINTY_MEASURE_WITH_UNIT (LENGTH_MEASURE( 1.000000000000000082E-05 ), #12067, 'distance_accuracy_value', 'NONE');
#8294=ORIENTED_EDGE ( 'NONE', *, *, #8970, .F. ) ;
#8295=CARTESIAN_POINT ( 'NONE',  ( 28.99095782554747913, 92.47818727009294548, -1.000000000000000000 ) ) ;
#8301=AXIS2_PLACEMENT_3D ( 'NONE', #8994, #11020, #1811 ) ;
#8306=VERTEX_POINT ( 'NONE', #8830 ) ;
#8320=DIRECTION ( 'NONE',  ( 0.000000000000000000, -1.000000000000000000, 0.000000000000000000 ) ) ;
#8324=ORIENTED_EDGE ( 'NONE', *, *, #2258, .T. ) ;
#8330=EDGE_CURVE ( 'NONE', #5069, #10466, #11594, .T. ) ;
#8338=CARTESIAN_POINT ( 'NONE',  ( 6.626776019045581556, 99.74475042915889844, -3.000000000000000000 ) ) ;
#8347=DIRECTION ( 'NONE',  ( -1.000000000000000000, 0.000000000000000000, -0.000000000000000000 ) ) ;
#8352=PRODUCT ( 'conveyor wheel', 'conveyor wheel', '', ( #7260 ) ) ;
#8358=EDGE_CURVE ( 'NONE', #7336, #4743, #2889, .T. ) ;
#8368=VERTEX_POINT ( 'NONE', #9684 ) ;
#8370=DIRECTION ( 'NONE',  ( 0.000000000000000000, 0.000000000000000000, 1.000000000000000000 ) ) ;
#8383=ORIENTED_EDGE ( 'NONE', *, *, #12077, .F. ) ;
#8405=DIRECTION ( 'NONE',  ( 0.000000000000000000, 0.000000000000000000, 1.000000000000000000 ) ) ;
#8406=CARTESIAN_POINT ( 'NONE',  ( 35.00000000000000000, 90.00000000000000000, -0.9999999999999970024 ) ) ;
#8415=VECTOR ( 'NONE', #838, 1000.000000000000000 ) ;
#8416=LINE ( 'NONE', #3452, #77 ) ;
#8433=ADVANCED_FACE ( 'NONE', ( #111 ), #6075, .T. ) ;
#8435=LINE ( 'NONE', #10395, #10127 ) ;
#8438=CARTESIAN_POINT ( 'NONE',  ( 35.00000000000000000, 90.00000000000000000, -3.000000000000000000 ) ) ;
#8446=ORIENTED_EDGE ( 'NONE', *, *, #4252, .T. ) ;
#8457=AXIS2_PLACEMENT_3D ( 'NONE', #9, #6832, #6772 ) ;
#8478=VERTEX_POINT ( 'NONE', #9214 ) ;
#8488=AXIS2_PLACEMENT_3D ( 'NONE', #491, #7570, #4436 ) ;
#8496=VERTEX_POINT ( 'NONE', #11966 ) ;
#8513=ORIENTED_EDGE ( 'NONE', *, *, #11633, .F. ) ;
#8518=ORIENTED_EDGE ( 'NONE', *, *, #4557, .T. ) ;
#8527=AXIS2_PLACEMENT_3D ( 'NONE', #1324, #9047, #12130 ) ;
#8528=CARTESIAN_POINT ( 'NONE',  ( 72.83557806687970526, 62.54593364529978317, 1.000000000000003109 ) ) ;
#8530=EDGE_CURVE ( 'NONE', #1585, #10599, #10352, .T. ) ;
#8531=CARTESIAN_POINT ( 'NONE',  ( 35.00000000000000000, 90.00000000000000000, -3.000000000000000000 ) ) ;
#8536=CIRCLE ( 'NONE', #6227, 28.99999999999999289 ) ;
#8568=EDGE_CURVE ( 'NONE', #8022, #454, #94, .T. ) ;
#8577=ORIENTED_EDGE ( 'NONE', *, *, #7590, .T. ) ;
#8579=ORIENTED_EDGE ( 'NONE', *, *, #10942, .T. ) ;
#8602=CARTESIAN_POINT ( 'NONE',  ( 7.577945032559769700, 99.43561875886716450, 3.000000000000001332 ) ) ;
#8611=EDGE_CURVE ( 'NONE', #6279, #11952, #7428, .T. ) ;
#8625=DIRECTION ( 'NONE',  ( -0.000000000000000000, -0.000000000000000000, -1.000000000000000000 ) ) ;
#8648=ORIENTED_EDGE ( 'NONE', *, *, #6736, .F. ) ;
#8665=DIRECTION ( 'NONE',  ( 0.000000000000000000, 0.000000000000000000, -1.000000000000000000 ) ) ;
#8672=EDGE_CURVE ( 'NONE', #4270, #3017, #6464, .T. ) ;
#8674=AXIS2_PLACEMENT_3D ( 'NONE', #665, #1462, #3503 ) ;
#8681=DIRECTION ( 'NONE',  ( 0.000000000000000000, 0.000000000000000000, 1.000000000000000000 ) ) ;
#8682=DIRECTION ( 'NONE',  ( 0.000000000000000000, 0.000000000000000000, -1.000000000000000000 ) ) ;
#8701=EDGE_CURVE ( 'NONE', #8368, #7529, #8435, .T. ) ;
#8716=AXIS2_PLACEMENT_3D ( 'NONE', #5203, #1336, #9126 ) ;
#8729=ORIENTED_EDGE ( 'NONE', *, *, #7590, .F. ) ;
#8735=CARTESIAN_POINT ( 'NONE',  ( 35.00000000000000000, 90.00000000000000000, 1.000000000000003553 ) ) ;
#8738=ADVANCED_FACE ( 'NONE', ( #12806 ), #4831, .T. ) ;
#8765=ORIENTED_EDGE ( 'NONE', *, *, #10673, .F. ) ;
#8768=VECTOR ( 'NONE', #7870, 1000.000000000000000 ) ;
#8779=DIRECTION ( 'NONE',  ( -0.000000000000000000, -0.000000000000000000, -1.000000000000000000 ) ) ;
#8793=EDGE_CURVE ( 'NONE', #7791, #1672, #5676, .T. ) ;
#8800=CARTESIAN_POINT ( 'NONE',  ( 52.44898870156725224, 66.83414752204051013, -1.000000000000000222 ) ) ;
#8812=LINE ( 'NONE', #12012, #6642 ) ;
#8816=ORIENTED_EDGE ( 'NONE', *, *, #11102, .T. ) ;
#8821=ORIENTED_EDGE ( 'NONE', *, *, #11796, .T. ) ;
#8830=CARTESIAN_POINT ( 'NONE',  ( 9.136132550659251450, 74.79933025939541835, 1.000000000000003553 ) ) ;
#8842=VECTOR ( 'NONE', #7898, 999.9999999999998863 ) ;
#8843=ADVANCED_FACE ( 'NONE', ( #4706 ), #3727, .F. ) ;
#8851=DIRECTION ( 'NONE',  ( -0.000000000000000000, 0.000000000000000000, 1.000000000000000000 ) ) ;
#8860=ORIENTED_EDGE ( 'NONE', *, *, #539, .F. ) ;
#8864=CARTESIAN_POINT ( 'NONE',  ( 7.266925300896119211, 98.48530999652632545, 4.000000000000000000 ) ) ;
#8872=CYLINDRICAL_SURFACE ( 'NONE', #8301, 28.99999999999999289 ) ;
#8875=CARTESIAN_POINT ( 'NONE',  ( 16.96438320935645905, 66.02675393316422969, 1.000000000000003109 ) ) ;
#8887=EDGE_LOOP ( 'NONE', ( #2831, #2953, #12877, #10841 ) ) ;
#8897=VECTOR ( 'NONE', #10814, 1000.000000000000114 ) ;
#8904=CARTESIAN_POINT ( 'NONE',  ( 17.54971918633085437, 66.83239978927272773, 4.000000000000000000 ) ) ;
#8914=VERTEX_POINT ( 'NONE', #10365 ) ;
#8916=ADVANCED_FACE ( 'NONE', ( #11278 ), #1268, .F. ) ;
#8917=ORIENTED_EDGE ( 'NONE', *, *, #12833, .T. ) ;
#8927=CARTESIAN_POINT ( 'NONE',  ( 35.75000000000000711, 93.50000000000000000, -4.802775637732004554 ) ) ;
#8929=DIRECTION ( 'NONE',  ( 0.000000000000000000, 0.000000000000000000, 1.000000000000000000 ) ) ;
#8963=CARTESIAN_POINT ( 'NONE',  ( 62.73309762663101452, 98.48529854432332797, 1.000000000000003109 ) ) ;
#8970=EDGE_CURVE ( 'NONE', #36, #5609, #9249, .T. ) ;
#8976=DIRECTION ( 'NONE',  ( 0.000000000000000000, 0.000000000000000000, -1.000000000000000000 ) ) ;
#8988=PLANE ( 'NONE',  #11786 ) ;
#8994=CARTESIAN_POINT ( 'NONE',  ( 35.00000000000000000, 90.00000000000000000, 4.000000000000000000 ) ) ;
#8997=CARTESIAN_POINT ( 'NONE',  ( 0.000000000000000000, 0.000000000000000000, 0.000000000000000000 ) ) ;
#8998=CIRCLE ( 'NONE', #4418, 6.499999999999999112 ) ;
#8999=LINE ( 'NONE', #23, #10823 ) ;
#9016=ADVANCED_BREP_SHAPE_REPRESENTATION ( '', ( #7850, #5704 ), #2789 ) ;
#9045=VERTEX_POINT ( 'NONE', #12525 ) ;
#9047=DIRECTION ( 'NONE',  ( -0.000000000000000000, -0.000000000000000000, -1.000000000000000000 ) ) ;
#9052=EDGE_CURVE ( 'NONE', #7127, #8087, #536, .T. ) ;
#9056=DIRECTION ( 'NONE',  ( 0.5877852522924770229, 0.8090169943749445647, 0.000000000000000000 ) ) ;
#9060=ORIENTED_EDGE ( 'NONE', *, *, #10942, .F. ) ;
#9073=VERTEX_POINT ( 'NONE', #6496 ) ;
#9074=FACE_OUTER_BOUND ( 'NONE', #12679, .T. ) ;
#9075=EDGE_CURVE ( 'NONE', #11004, #8177, #12657, .T. ) ;
#9094=EDGE_CURVE ( 'NONE', #4025, #12399, #22, .T. ) ;
#9099=VECTOR ( 'NONE', #5587, 1000.000000000000000 ) ;
#9112=VECTOR ( 'NONE', #12411, 1000.000000000000000 ) ;
#9116=CARTESIAN_POINT ( 'NONE',  ( 5.000000000000007994, 90.00000000000000000, 4.000000000000000000 ) ) ;
#9118=DIRECTION ( 'NONE',  ( 0.000000000000000000, -0.000000000000000000, -1.000000000000000000 ) ) ;
#9126=DIRECTION ( 'NONE',  ( -1.000000000000000000, 0.000000000000000000, 0.000000000000000000 ) ) ;
#9142=CARTESIAN_POINT ( 'NONE',  ( 30.78620769635677235, 85.05086326499690585, -1.000000000000000000 ) ) ;
#9144=ADVANCED_FACE ( 'NONE', ( #3699 ), #4476, .T. ) ;
#9154=CARTESIAN_POINT ( 'NONE',  ( 35.00000000000000000, 90.00000000000000000, 4.000000000000000000 ) ) ;
#9167=VERTEX_POINT ( 'NONE', #11470 ) ;
#9181=LINE ( 'NONE', #2194, #2067 ) ;
#9183=DIRECTION ( 'NONE',  ( -0.8090169943749485615, 0.5877852522924716938, 0.000000000000000000 ) ) ;
#9189=CARTESIAN_POINT ( 'NONE',  ( 52.45028081366923089, 66.83239978927284142, 2.333333333333333481 ) ) ;
#9190=FACE_OUTER_BOUND ( 'NONE', #9233, .T. ) ;
#9196=EDGE_CURVE ( 'NONE', #7336, #8306, #8137, .T. ) ;
#9214=CARTESIAN_POINT ( 'NONE',  ( 65.00000000000000000, 90.00000000000000000, 4.000000000000000000 ) ) ;
#9233=EDGE_LOOP ( 'NONE', ( #8729, #510, #5566, #9898, #10413, #4626 ) ) ;
#9242=EDGE_CURVE ( 'NONE', #330, #8478, #1053, .T. ) ;
#9249=LINE ( 'NONE', #8148, #6689 ) ;
#9252=ADVANCED_FACE ( 'NONE', ( #989 ), #8000, .F. ) ;
#9257=EDGE_CURVE ( 'NONE', #7589, #7916, #7016, .T. ) ;
#9270=ORIENTED_EDGE ( 'NONE', *, *, #3830, .T. ) ;
#9277=ORIENTED_EDGE ( 'NONE', *, *, #2803, .T. ) ;
#9289=EDGE_LOOP ( 'NONE', ( #6167, #12228, #6985, #9989 ) ) ;
#9298=VERTEX_POINT ( 'NONE', #2048 ) ;
#9308=CARTESIAN_POINT ( 'NONE',  ( 34.25000000000000000, 92.49999999999998579, 4.000000000000000000 ) ) ;
#9315=ADVANCED_FACE ( 'NONE', ( #1791, #11858 ), #12780, .T. ) ;
#9316=EDGE_CURVE ( 'NONE', #4104, #1224, #5185, .T. ) ;
#9317=LINE ( 'NONE', #2387, #1976 ) ;
#9321=LINE ( 'NONE', #274, #521 ) ;
#9334=CARTESIAN_POINT ( 'NONE',  ( 35.00000000000000000, 90.00000000000000000, -1.000000000000000000 ) ) ;
#9341=ORIENTED_EDGE ( 'NONE', *, *, #11905, .T. ) ;
#9343=DIRECTION ( 'NONE',  ( -1.000000000000000000, 0.000000000000000000, 0.000000000000000000 ) ) ;
#9354=CARTESIAN_POINT ( 'NONE',  ( 65.00000000000000000, 117.5000000000001705, -0.9999999999999970024 ) ) ;
#9362=ORIENTED_EDGE ( 'NONE', *, *, #9052, .F. ) ;
#9371=DIRECTION ( 'NONE',  ( -1.000000000000000000, 0.000000000000000000, 0.000000000000000000 ) ) ;
#9379=DIRECTION ( 'NONE',  ( -0.000000000000000000, -0.000000000000000000, -1.000000000000000000 ) ) ;
#9381=AXIS2_PLACEMENT_3D ( 'NONE', #5743, #4768, #10840 ) ;
#9389=EDGE_LOOP ( 'NONE', ( #7023, #9860, #2051, #7495 ) ) ;
#9394=DIRECTION ( 'NONE',  ( -0.000000000000000000, -1.000000000000000000, 0.000000000000000000 ) ) ;
#9398=ORIENTED_EDGE ( 'NONE', *, *, #3554, .F. ) ;
#9407=VECTOR ( 'NONE', #3251, 1000.000000000000000 ) ;
#9415=ORIENTED_EDGE ( 'NONE', *, *, #3609, .T. ) ;
#9420=CARTESIAN_POINT ( 'NONE',  ( 41.46432142674534305, 60.70473504998254555, -0.9999999999999970024 ) ) ;
#9443=CARTESIAN_POINT ( 'NONE',  ( 13.95244456248789788, 109.9499476216067819, -1.000000000000000000 ) ) ;
#9452=DIRECTION ( 'NONE',  ( -1.000000000000000000, 0.000000000000000000, 0.000000000000000000 ) ) ;
#9456=LINE ( 'NONE', #1853, #5764 ) ;
#9464=LINE ( 'NONE', #10384, #9112 ) ;
#9465=ORIENTED_EDGE ( 'NONE', *, *, #10006, .F. ) ;
#9469=CARTESIAN_POINT ( 'NONE',  ( 35.00000000000000000, 90.00000000000000000, 4.000000000000000000 ) ) ;
#9470=CARTESIAN_POINT ( 'NONE',  ( 35.49999999999993605, 122.5000000000000142, 1.000000000000003109 ) ) ;
#9471=VERTEX_POINT ( 'NONE', #1255 ) ;
#9482=DIRECTION ( 'NONE',  ( -0.000000000000000000, -0.000000000000000000, 1.000000000000000000 ) ) ;
#9483=ORIENTED_EDGE ( 'NONE', *, *, #11995, .T. ) ;
#9491=STYLED_ITEM('',(#13016),#7850);
#9522=CARTESIAN_POINT ( 'NONE',  ( 35.00000000000000000, 90.00000000000000000, -0.9999999999999970024 ) ) ;
#9524=CARTESIAN_POINT ( 'NONE',  ( 43.71630314554308683, 62.34089554097971586, -0.9999999999999970024 ) ) ;
#9527=DIRECTION ( 'NONE',  ( -0.000000000000000000, -0.000000000000000000, -1.000000000000000000 ) ) ;
#9530=AXIS2_PLACEMENT_3D ( 'NONE', #6920, #9929, #6857 ) ;
#9539=ORIENTED_EDGE ( 'NONE', *, *, #2241, .F. ) ;
#9542=DIRECTION ( 'NONE',  ( 3.497202527569242313E-15, -1.000000000000000000, 0.000000000000000000 ) ) ;
#9544=ORIENTED_EDGE ( 'NONE', *, *, #2258, .F. ) ;
#9547=CARTESIAN_POINT ( 'NONE',  ( 35.49999999999995026, 119.9958330439412890, -3.000000000000000000 ) ) ;
#9561=ORIENTED_EDGE ( 'NONE', *, *, #6736, .T. ) ;
#9565=ORIENTED_EDGE ( 'NONE', *, *, #1250, .F. ) ;
#9578=DIRECTION ( 'NONE',  ( -0.000000000000000000, 0.000000000000000000, 1.000000000000000000 ) ) ;
#9590=ADVANCED_FACE ( 'NONE', ( #4595 ), #2635, .T. ) ;
#9597=LINE ( 'NONE', #12674, #5437 ) ;
#9615=EDGE_CURVE ( 'NONE', #955, #10005, #3686, .T. ) ;
#9621=CIRCLE ( 'NONE', #3982, 28.99999999999999289 ) ;
#9623=UNCERTAINTY_MEASURE_WITH_UNIT (LENGTH_MEASURE( 1.000000000000000082E-05 ), #10017, 'distance_accuracy_value', 'NONE');
#9626=EDGE_CURVE ( 'NONE', #9895, #11248, #6483, .T. ) ;
#9644=CIRCLE ( 'NONE', #2760, 28.99999999999999289 ) ;
#9651=CARTESIAN_POINT ( 'NONE',  ( 4.245171717594923066, 100.5185805753332033, 1.000000000000003109 ) ) ;
#9654=EDGE_LOOP ( 'NONE', ( #5611, #3605, #7574, #8860 ) ) ;
#9672=LINE ( 'NONE', #5482, #10548 ) ;
#9673=CARTESIAN_POINT ( 'NONE',  ( 35.00000000000000000, 90.00000000000000000, 22.38477631085024555 ) ) ;
#9674=ORIENTED_EDGE ( 'NONE', *, *, #7629, .F. ) ;
#9684=CARTESIAN_POINT ( 'NONE',  ( 62.42406877266672183, 99.43633196372844907, 4.000000000000000000 ) ) ;
#9685=ORIENTED_EDGE ( 'NONE', *, *, #3580, .F. ) ;
#9691=DIRECTION ( 'NONE',  ( 1.000000000000000000, 2.135044278125301343E-15, 0.000000000000000000 ) ) ;
#9692=AXIS2_PLACEMENT_3D ( 'NONE', #2279, #10310, #4239 ) ;
#9703=CARTESIAN_POINT ( 'NONE',  ( 35.00000000000000000, 90.00000000000000000, 22.38477631085024555 ) ) ;
#9744=FACE_OUTER_BOUND ( 'NONE', #7394, .T. ) ;
#9762=CARTESIAN_POINT ( 'NONE',  ( 72.83557806687970526, 62.54593364529978317, 1.000000000000003109 ) ) ;
#9767=DIRECTION ( 'NONE',  ( -1.000000000000000000, 0.000000000000000000, -0.000000000000000000 ) ) ;
#9783=CARTESIAN_POINT ( 'NONE',  ( 35.49951382533862443, 118.9974510565036070, 4.000000000000000000 ) ) ;
#9786=CARTESIAN_POINT ( 'NONE',  ( 44.20597631976078645, 117.5000000000000568, 1.000000000000003109 ) ) ;
#9808=CARTESIAN_POINT ( 'NONE',  ( 35.00000000000000000, 90.00000000000000000, 4.000000000000000000 ) ) ;
#9813=ORIENTED_EDGE ( 'NONE', *, *, #4154, .F. ) ;
#9826=ADVANCED_FACE ( 'NONE', ( #11764 ), #11892, .T. ) ;
#9829=CARTESIAN_POINT ( 'NONE',  ( 35.00000000000000000, 90.00000000000000000, 4.000000000000000000 ) ) ;
#9835=CARTESIAN_POINT ( 'NONE',  ( 34.25000000000000000, 93.50000000000000000, -3.000000000000000000 ) ) ;
#9844=CARTESIAN_POINT ( 'NONE',  ( 7.264852530253062213, 98.48596457872582732, 0.6666666666666654084 ) ) ;
#9845=VECTOR ( 'NONE', #3290, 1000.000000000000000 ) ;
#9850=ORIENTED_EDGE ( 'NONE', *, *, #5381, .T. ) ;
#9860=ORIENTED_EDGE ( 'NONE', *, *, #1029, .F. ) ;
#9861=PLANE ( 'NONE',  #8054 ) ;
#9866=VERTEX_POINT ( 'NONE', #5811 ) ;
#9867=ORIENTED_EDGE ( 'NONE', *, *, #6025, .T. ) ;
#9875=ORIENTED_EDGE ( 'NONE', *, *, #7411, .T. ) ;
#9879=EDGE_LOOP ( 'NONE', ( #9960, #9277, #11561, #10544 ) ) ;
#9893=AXIS2_PLACEMENT_3D ( 'NONE', #6056, #3789, #7768 ) ;
#9895=VERTEX_POINT ( 'NONE', #4834 ) ;
#9896=DIRECTION ( 'NONE',  ( 1.914177628664063178E-15, -1.000000000000000000, 0.000000000000000000 ) ) ;
#9898=ORIENTED_EDGE ( 'NONE', *, *, #5548, .T. ) ;
#9903=CIRCLE ( 'NONE', #6979, 30.00000000000000000 ) ;
#9908=DIRECTION ( 'NONE',  ( 0.8090169943749456749, -0.5877852522924754686, 0.000000000000000000 ) ) ;
#9910=EDGE_CURVE ( 'NONE', #1278, #1585, #7649, .T. ) ;
#9911=LINE ( 'NONE', #942, #10034 ) ;
#9912=VECTOR ( 'NONE', #737, 1000.000000000000000 ) ;
#9918=DIRECTION ( 'NONE',  ( -1.000000000000000000, 0.000000000000000000, 0.000000000000000000 ) ) ;
#9929=DIRECTION ( 'NONE',  ( 0.000000000000000000, 0.000000000000000000, -1.000000000000000000 ) ) ;
#9960=ORIENTED_EDGE ( 'NONE', *, *, #1029, .T. ) ;
#9972=DIRECTION ( 'NONE',  ( -0.000000000000000000, 0.000000000000000000, -1.000000000000000000 ) ) ;
#9984=DIRECTION ( 'NONE',  ( 0.000000000000000000, 0.000000000000000000, 1.000000000000000000 ) ) ;
#9989=ORIENTED_EDGE ( 'NONE', *, *, #3757, .F. ) ;
#9992=DIRECTION ( 'NONE',  ( 0.000000000000000000, 0.000000000000000000, 1.000000000000000000 ) ) ;
#10000=FACE_OUTER_BOUND ( 'NONE', #1499, .T. ) ;
#10003=EDGE_LOOP ( 'NONE', ( #1889, #5985, #4064, #10058, #3344, #12295 ) ) ;
#10005=VERTEX_POINT ( 'NONE', #3269 ) ;
#10006=EDGE_CURVE ( 'NONE', #3338, #6015, #2927, .T. ) ;
#10017=( LENGTH_UNIT ( ) NAMED_UNIT ( * ) SI_UNIT ( .MILLI., .METRE. ) );
#10027=ORIENTED_EDGE ( 'NONE', *, *, #11102, .F. ) ;
#10028=DIRECTION ( 'NONE',  ( 0.5877852522924726930, -0.8090169943749476733, -0.000000000000000000 ) ) ;
#10030=EDGE_LOOP ( 'NONE', ( #4482, #11686, #10200, #434, #1759, #5502 ) ) ;
#10034=VECTOR ( 'NONE', #8929, 1000.000000000000000 ) ;
#10044=CARTESIAN_POINT ( 'NONE',  ( 62.42613047537196991, 99.43702109502110886, 2.333333333333333481 ) ) ;
#10055=ORIENTED_EDGE ( 'NONE', *, *, #10889, .T. ) ;
#10058=ORIENTED_EDGE ( 'NONE', *, *, #6879, .T. ) ;
#10068=FACE_BOUND ( 'NONE', #6722, .T. ) ;
#10069=EDGE_CURVE ( 'NONE', #12641, #12892, #5995, .T. ) ;
#10072=CARTESIAN_POINT ( 'NONE',  ( 62.73102604205943322, 98.48470356904833523, 2.000000000000001776 ) ) ;
#10086=CARTESIAN_POINT ( 'NONE',  ( 18.35999867260799689, 66.24638416932324958, -1.000000000000000000 ) ) ;
#10092=DIRECTION ( 'NONE',  ( -0.9510565162951529761, -0.3090169943749492276, 0.000000000000000000 ) ) ;
#10100=CARTESIAN_POINT ( 'NONE',  ( 17.55170909815984004, 66.83416404266884570, 4.000000000000000000 ) ) ;
#10126=ORIENTED_EDGE ( 'NONE', *, *, #9257, .T. ) ;
#10127=VECTOR ( 'NONE', #12561, 1000.000000000000114 ) ;
#10128=ORIENTED_EDGE ( 'NONE', *, *, #6342, .T. ) ;
#10130=ORIENTED_EDGE ( 'NONE', *, *, #8672, .F. ) ;
#10135=FACE_OUTER_BOUND ( 'NONE', #1055, .T. ) ;
#10147=EDGE_CURVE ( 'NONE', #8074, #454, #7504, .T. ) ;
#10156=ORIENTED_EDGE ( 'NONE', *, *, #8793, .F. ) ;
#10168=AXIS2_PLACEMENT_3D ( 'NONE', #10172, #4165, #10238 ) ;
#10172=CARTESIAN_POINT ( 'NONE',  ( 51.64126381929429499, 66.24461453698036451, 4.000000000000000000 ) ) ;
#10176=AXIS2_PLACEMENT_3D ( 'NONE', #2834, #10805, #7927 ) ;
#10181=CARTESIAN_POINT ( 'NONE',  ( 17.55231228847961944, 66.83584248194507893, 2.000000000000002220 ) ) ;
#10184=EDGE_CURVE ( 'NONE', #7916, #12941, #194, .T. ) ;
#10189=ORIENTED_EDGE ( 'NONE', *, *, #10929, .T. ) ;
#10200=ORIENTED_EDGE ( 'NONE', *, *, #5145, .F. ) ;
#10211=LINE ( 'NONE', #1047, #7268 ) ;
#10213=DIRECTION ( 'NONE',  ( 0.9510565162951543083, -0.3090169943749451198, 0.000000000000000000 ) ) ;
#10231=AXIS2_PLACEMENT_3D ( 'NONE', #5146, #7968, #12021 ) ;
#10238=DIRECTION ( 'NONE',  ( 0.5877852522924753575, -0.8090169943749457859, 0.000000000000000000 ) ) ;
#10248=AXIS2_PLACEMENT_3D ( 'NONE', #8202, #4405, #7218 ) ;
#10277=VECTOR ( 'NONE', #7118, 1000.000000000000114 ) ;
#10294=( NAMED_UNIT ( * ) PLANE_ANGLE_UNIT ( ) SI_UNIT ( $, .RADIAN. ) );
#10298=DIRECTION ( 'NONE',  ( -1.000000000000000000, -9.570888143320317860E-16, 0.000000000000000000 ) ) ;
#10310=DIRECTION ( 'NONE',  ( -0.8090169943749457859, -0.5877852522924753575, 0.000000000000000000 ) ) ;
#10311=EDGE_CURVE ( 'NONE', #8478, #6336, #6901, .T. ) ;
#10313=CARTESIAN_POINT ( 'NONE',  ( 52.22659979626836702, 65.43896868087158225, 1.000000000000003109 ) ) ;
#10347=ADVANCED_FACE ( 'NONE', ( #2669 ), #6645, .T. ) ;
#10352=CIRCLE ( 'NONE', #12655, 6.499999999999999112 ) ;
#10354=EDGE_CURVE ( 'NONE', #4104, #4463, #9597, .T. ) ;
#10365=CARTESIAN_POINT ( 'NONE',  ( 6.000000000000008882, 90.00000000000000000, 4.000000000000000000 ) ) ;
#10368=AXIS2_PLACEMENT_3D ( 'NONE', #6323, #7248, #12222 ) ;
#10373=ORIENTED_EDGE ( 'NONE', *, *, #9075, .T. ) ;
#10375=CIRCLE ( 'NONE', #8083, 6.499999999999999112 ) ;
#10379=DIRECTION ( 'NONE',  ( 0.000000000000000000, 0.000000000000000000, -1.000000000000000000 ) ) ;
#10384=CARTESIAN_POINT ( 'NONE',  ( 28.68194083117252902, 91.52713075379780605, 22.38477631085024555 ) ) ;
#10386=VECTOR ( 'NONE', #279, 1000.000000000000000 ) ;
#10391=CARTESIAN_POINT ( 'NONE',  ( 34.49999999999998579, 96.48074069840785683, 4.000000000000000000 ) ) ;
#10392=ORIENTED_EDGE ( 'NONE', *, *, #2366, .T. ) ;
#10395=CARTESIAN_POINT ( 'NONE',  ( 62.42613047537196991, 99.43702109502110886, 4.000000000000000000 ) ) ;
#10403=VERTEX_POINT ( 'NONE', #9786 ) ;
#10412=CARTESIAN_POINT ( 'NONE',  ( 39.21379230364324542, 85.05086326499692007, -0.9999999999999970024 ) ) ;
#10413=ORIENTED_EDGE ( 'NONE', *, *, #9316, .F. ) ;
#10425=DIRECTION ( 'NONE',  ( -0.9510565162951543083, 0.3090169943749451198, 0.000000000000000000 ) ) ;
#10427=CARTESIAN_POINT ( 'NONE',  ( 17.26299177799148055, 43.12143982588584379, -0.9999999999999970024 ) ) ;
#10429=DIRECTION ( 'NONE',  ( 1.000000000000000000, 1.914177628664063178E-15, -0.000000000000000000 ) ) ;
#10434=VERTEX_POINT ( 'NONE', #814 ) ;
#10446=CARTESIAN_POINT ( 'NONE',  ( 12.55092940903992549, 109.9007343985615393, -3.000000000000000000 ) ) ;
#10461=ORIENTED_EDGE ( 'NONE', *, *, #1979, .F. ) ;
#10466=VERTEX_POINT ( 'NONE', #5914 ) ;
#10477=DIRECTION ( 'NONE',  ( -0.000000000000000000, -1.000000000000000000, 0.000000000000000000 ) ) ;
#10483=LINE ( 'NONE', #11596, #6609 ) ;
#10501=FILL_AREA_STYLE ('',( #11481 ) ) ;
#10502=AXIS2_PLACEMENT_3D ( 'NONE', #11839, #10974, #1093 ) ;
#10513=EDGE_CURVE ( 'NONE', #8267, #1018, #9911, .T. ) ;
#10514=ORIENTED_EDGE ( 'NONE', *, *, #1524, .F. ) ;
#10516=ORIENTED_EDGE ( 'NONE', *, *, #6307, .F. ) ;
#10518=CARTESIAN_POINT ( 'NONE',  ( 30.78620769635677590, 85.05086326499690585, 4.000000000000000000 ) ) ;
#10532=CARTESIAN_POINT ( 'NONE',  ( 5.000000000000007994, 90.00000000000000000, -3.000000000000000000 ) ) ;
#10539=AXIS2_PLACEMENT_3D ( 'NONE', #3634, #10429, #1598 ) ;
#10541=AXIS2_PLACEMENT_3D ( 'NONE', #2728, #7498, #1537 ) ;
#10544=ORIENTED_EDGE ( 'NONE', *, *, #5548, .F. ) ;
#10548=VECTOR ( 'NONE', #2618, 1000.000000000000114 ) ;
#10555=CARTESIAN_POINT ( 'NONE',  ( 35.00000000000000000, 90.00000000000000000, 22.38477631085024555 ) ) ;
#10562=CARTESIAN_POINT ( 'NONE',  ( 7.577945032559769700, 99.43561875886716450, 2.000000000000002665 ) ) ;
#10563=FACE_OUTER_BOUND ( 'NONE', #2601, .T. ) ;
#10589=DIRECTION ( 'NONE',  ( 0.000000000000000000, 0.000000000000000000, -1.000000000000000000 ) ) ;
#10599=VERTEX_POINT ( 'NONE', #6902 ) ;
#10600=ORIENTED_EDGE ( 'NONE', *, *, #9094, .F. ) ;
#10602=CARTESIAN_POINT ( 'NONE',  ( 7.575919367743916943, 99.43635506061835372, 1.000000000000003109 ) ) ;
#10616=DIRECTION ( 'NONE',  ( -1.000000000000000000, 0.000000000000000000, 0.000000000000000000 ) ) ;
#10619=EDGE_CURVE ( 'NONE', #7663, #619, #3818, .T. ) ;
#10623=DIRECTION ( 'NONE',  ( 0.000000000000000000, 0.000000000000000000, 1.000000000000000000 ) ) ;
#10640=CARTESIAN_POINT ( 'NONE',  ( 35.00000000000000000, 90.00000000000000000, 22.38477631085024555 ) ) ;
#10641=DIRECTION ( 'NONE',  ( 0.000000000000000000, 0.000000000000000000, -1.000000000000000000 ) ) ;
#10646=FACE_OUTER_BOUND ( 'NONE', #3668, .T. ) ;
#10672=VECTOR ( 'NONE', #3172, 1000.000000000000000 ) ;
#10673=EDGE_CURVE ( 'NONE', #9073, #6886, #9621, .T. ) ;
#10676=EDGE_CURVE ( 'NONE', #10005, #12318, #11216, .T. ) ;
#10677=LINE ( 'NONE', #8528, #3798 ) ;
#10678=CARTESIAN_POINT ( 'NONE',  ( 31.59522469073172601, 84.46307801270442894, 4.000000000000000000 ) ) ;
#10707=DIRECTION ( 'NONE',  ( -1.000000000000000000, 0.000000000000000000, 0.000000000000000000 ) ) ;
#10708=DIRECTION ( 'NONE',  ( -1.000000000000000000, 0.000000000000000000, 0.000000000000000000 ) ) ;
#10792=CARTESIAN_POINT ( 'NONE',  ( 35.00000000000000000, 90.00000000000000000, -1.000000000000000000 ) ) ;
#10805=DIRECTION ( 'NONE',  ( 0.000000000000000000, 0.000000000000000000, -1.000000000000000000 ) ) ;
#10806=DIRECTION ( 'NONE',  ( -0.3090169943749500048, 0.9510565162951528650, 0.000000000000000000 ) ) ;
#10810=DIRECTION ( 'NONE',  ( -1.000000000000000000, -9.570888143320317860E-16, 0.000000000000000000 ) ) ;
#10814=DIRECTION ( 'NONE',  ( -0.9510565162951533091, -0.3090169943749480619, 0.000000000000000000 ) ) ;
#10817=CARTESIAN_POINT ( 'NONE',  ( 7.576448291486922670, 99.43666122937791840, 4.000000000000000000 ) ) ;
#10821=EDGE_LOOP ( 'NONE', ( #1638, #7849, #9685, #5038 ) ) ;
#10823=VECTOR ( 'NONE', #822, 1000.000000000000000 ) ;
#10840=DIRECTION ( 'NONE',  ( -1.000000000000000000, 0.000000000000000000, -0.000000000000000000 ) ) ;
#10841=ORIENTED_EDGE ( 'NONE', *, *, #10069, .T. ) ;
#10843=DIRECTION ( 'NONE',  ( -1.000000000000000000, 0.000000000000000000, 0.000000000000000000 ) ) ;
#10845=VECTOR ( 'NONE', #7549, 1000.000000000000227 ) ;
#10852=DIRECTION ( 'NONE',  ( -5.551115123125781124E-15, 1.000000000000000000, 0.000000000000000000 ) ) ;
#10854=AXIS2_PLACEMENT_3D ( 'NONE', #11983, #3891, #3030 ) ;
#10865=LINE ( 'NONE', #8904, #1191 ) ;
#10875=ORIENTED_EDGE ( 'NONE', *, *, #11995, .F. ) ;
#10876=DIRECTION ( 'NONE',  ( -1.000000000000000000, 1.387778780781446938E-14, 0.000000000000000000 ) ) ;
#10882=CIRCLE ( 'NONE', #2742, 6.499999999999999112 ) ;
#10889=EDGE_CURVE ( 'NONE', #9045, #4210, #417, .T. ) ;
#10910=PLANE ( 'NONE',  #6733 ) ;
#10929=EDGE_CURVE ( 'NONE', #1906, #5609, #133, .T. ) ;
#10942=EDGE_CURVE ( 'NONE', #11004, #4871, #7749, .T. ) ;
#10974=DIRECTION ( 'NONE',  ( 0.3090169943749492276, -0.9510565162951530871, 0.000000000000000000 ) ) ;
#10983=ORIENTED_EDGE ( 'NONE', *, *, #4213, .T. ) ;
#10985=CARTESIAN_POINT ( 'NONE',  ( 62.73303611935715196, 98.48533184915085315, 4.000000000000000000 ) ) ;
#10990=EDGE_CURVE ( 'NONE', #4210, #9471, #2120, .T. ) ;
#11000=EDGE_LOOP ( 'NONE', ( #11589, #10126, #8094, #9362 ) ) ;
#11004=VERTEX_POINT ( 'NONE', #10086 ) ;
#11005=ADVANCED_FACE ( 'NONE', ( #5967 ), #928, .T. ) ;
#11012=CARTESIAN_POINT ( 'NONE',  ( 41.46432142674534305, 60.70473504998254555, 1.000000000000003553 ) ) ;
#11020=DIRECTION ( 'NONE',  ( -0.000000000000000000, -0.000000000000000000, -1.000000000000000000 ) ) ;
#11023=CARTESIAN_POINT ( 'NONE',  ( 11.38811426945699701, 73.16316976839823383, 4.000000000000000000 ) ) ;
#11043=DIRECTION ( 'NONE',  ( 0.000000000000000000, 0.000000000000000000, -1.000000000000000000 ) ) ;
#11069=CARTESIAN_POINT ( 'NONE',  ( 35.00000000000000000, 90.00000000000000000, -1.000000000000000000 ) ) ;
#11102=EDGE_CURVE ( 'NONE', #5885, #9895, #6698, .T. ) ;
#11105=ORIENTED_EDGE ( 'NONE', *, *, #10184, .T. ) ;
#11124=EDGE_LOOP ( 'NONE', ( #10027, #68, #10055, #5622 ) ) ;
#11126=LINE ( 'NONE', #6158, #11795 ) ;
#11131=CIRCLE ( 'NONE', #3427, 0.9999999999999991118 ) ;
#11137=DIRECTION ( 'NONE',  ( 0.000000000000000000, 0.000000000000000000, 1.000000000000000000 ) ) ;
#11157=FACE_OUTER_BOUND ( 'NONE', #199, .T. ) ;
#11158=CARTESIAN_POINT ( 'NONE',  ( 65.00000000000000000, 90.00000000000000000, 1.000000000000003553 ) ) ;
#11160=ORIENTED_EDGE ( 'NONE', *, *, #9257, .F. ) ;
#11164=CIRCLE ( 'NONE', #8047, 28.99999999999999289 ) ;
#11166=DIRECTION ( 'NONE',  ( 0.000000000000000000, 0.000000000000000000, -1.000000000000000000 ) ) ;
#11168=CARTESIAN_POINT ( 'NONE',  ( 17.55098605904792564, 66.83414348997642662, 1.000000000000003109 ) ) ;
#11169=ORIENTED_EDGE ( 'NONE', *, *, #8611, .T. ) ;
#11170=EDGE_CURVE ( 'NONE', #9866, #8130, #331, .T. ) ;
#11175=AXIS2_PLACEMENT_3D ( 'NONE', #828, #6721, #2681 ) ;
#11184=PLANE ( 'NONE',  #7797 ) ;
#11203=DIRECTION ( 'NONE',  ( 0.000000000000000000, 0.000000000000000000, 1.000000000000000000 ) ) ;
#11207=AXIS2_PLACEMENT_3D ( 'NONE', #610, #7554, #8347 ) ;
#11213=CARTESIAN_POINT ( 'NONE',  ( 41.46432142674534305, 60.70473504998254555, -3.000000000000000000 ) ) ;
#11216=LINE ( 'NONE', #344, #9407 ) ;
#11224=CARTESIAN_POINT ( 'NONE',  ( 35.49999999999995026, 119.9958330439412890, -0.9999999999999970024 ) ) ;
#11236=VERTEX_POINT ( 'NONE', #4214 ) ;
#11248=VERTEX_POINT ( 'NONE', #9308 ) ;
#11255=LINE ( 'NONE', #3025, #11896 ) ;
#11272=EDGE_CURVE ( 'NONE', #12892, #9866, #10882, .T. ) ;
#11273=CARTESIAN_POINT ( 'NONE',  ( 64.85903780527353035, 87.09520029206045422, -0.9999999999999970024 ) ) ;
#11278=FACE_OUTER_BOUND ( 'NONE', #2631, .T. ) ;
#11283=ORIENTED_EDGE ( 'NONE', *, *, #9316, .T. ) ;
#11288=DIRECTION ( 'NONE',  ( 0.9510565162951530871, 0.3090169943749492276, 0.000000000000000000 ) ) ;
#11291=AXIS2_PLACEMENT_3D ( 'NONE', #11069, #5052, #4993 ) ;
#11296=CARTESIAN_POINT ( 'NONE',  ( 65.00000000000000000, 90.00000000000000000, -3.000000000000000000 ) ) ;
#11307=ORIENTED_EDGE ( 'NONE', *, *, #462, .F. ) ;
#11310=ORIENTED_EDGE ( 'NONE', *, *, #663, .T. ) ;
#11327=ORIENTED_EDGE ( 'NONE', *, *, #4154, .T. ) ;
#11341=EDGE_CURVE ( 'NONE', #4076, #10466, #10677, .T. ) ;
#11347=ORIENTED_EDGE ( 'NONE', *, *, #4582, .F. ) ;
#11349=AXIS2_PLACEMENT_3D ( 'NONE', #353, #12213, #11288 ) ;
#11360=EDGE_LOOP ( 'NONE', ( #11105, #3924, #8816, #8250, #10514, #4823 ) ) ;
#11367=ORIENTED_EDGE ( 'NONE', *, *, #10619, .T. ) ;
#11371=ORIENTED_EDGE ( 'NONE', *, *, #364, .T. ) ;
#11396=CARTESIAN_POINT ( 'NONE',  ( 28.50000000000000355, 90.00000000000000000, 22.38477631085024555 ) ) ;
#11398=ADVANCED_FACE ( 'NONE', ( #7604 ), #7540, .T. ) ;
#11403=VECTOR ( 'NONE', #8092, 1000.000000000000227 ) ;
#11406=CARTESIAN_POINT ( 'NONE',  ( 7.575919367743916943, 99.43635506061835372, 1.000000000000003109 ) ) ;
#11409=CIRCLE ( 'NONE', #5773, 28.99999999999999289 ) ;
#11414=CARTESIAN_POINT ( 'NONE',  ( 35.00000000000000000, 90.00000000000000000, -1.000000000000000000 ) ) ;
#11423=EDGE_LOOP ( 'NONE', ( #8294, #11347, #10130, #9867, #5231, #10189 ) ) ;
#11429=VERTEX_POINT ( 'NONE', #4665 ) ;
#11430=DIRECTION ( 'NONE',  ( -0.000000000000000000, -0.000000000000000000, -1.000000000000000000 ) ) ;
#11469=EDGE_CURVE ( 'NONE', #9298, #5069, #2686, .T. ) ;
#11470=CARTESIAN_POINT ( 'NONE',  ( 18.35999869903453430, 66.24638416994363865, 4.000000000000000000 ) ) ;
#11481=FILL_AREA_STYLE_COLOUR ( '', #684 ) ;
#11486=CARTESIAN_POINT ( 'NONE',  ( 35.49992570027444572, 118.9956906159209069, 3.000000000000000888 ) ) ;
#11491=DIRECTION ( 'NONE',  ( 0.000000000000000000, -0.000000000000000000, -1.000000000000000000 ) ) ;
#11503=EDGE_LOOP ( 'NONE', ( #6482, #6937, #4399, #5096, #7891, #2029, #2272, #984 ) ) ;
#11526=EDGE_LOOP ( 'NONE', ( #894, #1165, #4461, #11367 ) ) ;
#11533=LINE ( 'NONE', #2649, #12309 ) ;
#11547=PRESENTATION_STYLE_ASSIGNMENT (( #7560 ) ) ;
#11548=VECTOR ( 'NONE', #1688, 1000.000000000000227 ) ;
#11561=ORIENTED_EDGE ( 'NONE', *, *, #4252, .F. ) ;
#11563=EDGE_CURVE ( 'NONE', #12318, #1018, #8998, .T. ) ;
#11570=ORIENTED_EDGE ( 'NONE', *, *, #596, .T. ) ;
#11581=LINE ( 'NONE', #6540, #12708 ) ;
#11589=ORIENTED_EDGE ( 'NONE', *, *, #5470, .F. ) ;
#11594=CIRCLE ( 'NONE', #5942, 28.99999999999999289 ) ;
#11596=CARTESIAN_POINT ( 'NONE',  ( 52.22659979626835991, 65.43896868087158225, -3.000000000000000000 ) ) ;
#11607=CARTESIAN_POINT ( 'NONE',  ( 7.573869524628007888, 99.43702109502098097, 4.000000000000000000 ) ) ;
#11617=AXIS2_PLACEMENT_3D ( 'NONE', #5716, #8976, #12846 ) ;
#11633=EDGE_CURVE ( 'NONE', #4210, #9895, #5168, .T. ) ;
#11651=ORIENTED_EDGE ( 'NONE', *, *, #2803, .F. ) ;
#11664=VECTOR ( 'NONE', #9542, 1000.000000000000000 ) ;
#11671=ORIENTED_EDGE ( 'NONE', *, *, #10676, .F. ) ;
#11674=ADVANCED_FACE ( 'NONE', ( #4264 ), #4199, .F. ) ;
#11685=DIRECTION ( 'NONE',  ( -1.000000000000000000, -5.551115123125781124E-15, 0.000000000000000000 ) ) ;
#11686=ORIENTED_EDGE ( 'NONE', *, *, #4700, .T. ) ;
#11688=VERTEX_POINT ( 'NONE', #2365 ) ;
#11697=CARTESIAN_POINT ( 'NONE',  ( 34.50001867552290946, 118.9978264099154615, 4.000000000000000000 ) ) ;
#11743=DIRECTION ( 'NONE',  ( -1.000000000000000000, 0.000000000000000000, 0.000000000000000000 ) ) ;
#11764=FACE_OUTER_BOUND ( 'NONE', #4166, .T. ) ;
#11769=DIRECTION ( 'NONE',  ( 0.000000000000000000, 0.000000000000000000, 1.000000000000000000 ) ) ;
#11771=DIRECTION ( 'NONE',  ( -0.000000000000000000, -0.000000000000000000, 1.000000000000000000 ) ) ;
#11775=VERTEX_POINT ( 'NONE', #9420 ) ;
#11786=AXIS2_PLACEMENT_3D ( 'NONE', #8927, #7817, #4940 ) ;
#11795=VECTOR ( 'NONE', #5355, 1000.000000000000000 ) ;
#11796=EDGE_CURVE ( 'NONE', #3150, #8914, #9644, .T. ) ;
#11797=CARTESIAN_POINT ( 'NONE',  ( 51.63935276957964504, 66.24642824321904300, 4.000000000000000000 ) ) ;
#11807=CARTESIAN_POINT ( 'NONE',  ( 35.00000000000000000, 90.00000000000000000, 4.000000000000000000 ) ) ;
#11823=CIRCLE ( 'NONE', #7012, 6.499999999999999112 ) ;
#11826=LINE ( 'NONE', #12874, #8842 ) ;
#11836=ORIENTED_EDGE ( 'NONE', *, *, #3026, .T. ) ;
#11839=CARTESIAN_POINT ( 'NONE',  ( 62.73514746974691292, 98.48596457872595522, 4.000000000000000000 ) ) ;
#11846=ORIENTED_EDGE ( 'NONE', *, *, #9910, .F. ) ;
#11854=DIRECTION ( 'NONE',  ( 0.000000000000000000, 0.000000000000000000, 1.000000000000000000 ) ) ;
#11858=FACE_OUTER_BOUND ( 'NONE', #3102, .T. ) ;
#11871=AXIS2_PLACEMENT_3D ( 'NONE', #2562, #4329, #7464 ) ;
#11872=ADVANCED_FACE ( 'NONE', ( #9744 ), #12814, .F. ) ;
#11892=CYLINDRICAL_SURFACE ( 'NONE', #3356, 6.499999999999999112 ) ;
#11896=VECTOR ( 'NONE', #10213, 1000.000000000000000 ) ;
#11901=VECTOR ( 'NONE', #6789, 1000.000000000000000 ) ;
#11905=EDGE_CURVE ( 'NONE', #9298, #12318, #12534, .T. ) ;
#11907=ADVANCED_FACE ( 'NONE', ( #8104 ), #476, .T. ) ;
#11912=AXIS2_PLACEMENT_3D ( 'NONE', #10640, #4694, #7821 ) ;
#11913=DIRECTION ( 'NONE',  ( 1.000000000000000000, -6.405132834375904028E-15, 0.000000000000000000 ) ) ;
#11935=CARTESIAN_POINT ( 'NONE',  ( 7.264852530253062213, 98.48596457872582732, 2.333333333333333037 ) ) ;
#11940=VERTEX_POINT ( 'NONE', #11168 ) ;
#11946=LINE ( 'NONE', #6975, #3635 ) ;
#11952=VERTEX_POINT ( 'NONE', #3512 ) ;
#11957=EDGE_LOOP ( 'NONE', ( #10373, #5537, #12664, #6412 ) ) ;
#11961=CARTESIAN_POINT ( 'NONE',  ( 35.00000000000000000, 90.00000000000000000, -3.000000000000000000 ) ) ;
#11966=CARTESIAN_POINT ( 'NONE',  ( 9.136132550659251450, 74.79933025939541835, -0.9999999999999970024 ) ) ;
#11981=ORIENTED_EDGE ( 'NONE', *, *, #1995, .T. ) ;
#11983=CARTESIAN_POINT ( 'NONE',  ( 35.00000000000000000, 90.00000000000000000, 4.000000000000000000 ) ) ;
#11995=EDGE_CURVE ( 'NONE', #8496, #4743, #442, .T. ) ;
#12001=CARTESIAN_POINT ( 'NONE',  ( 35.00000000000000000, 90.00000000000000000, -0.9999999999999970024 ) ) ;
#12003=DIRECTION ( 'NONE',  ( -1.000000000000000000, 0.000000000000000000, 0.000000000000000000 ) ) ;
#12006=PLANE ( 'NONE',  #10168 ) ;
#12009=CARTESIAN_POINT ( 'NONE',  ( 62.42406877266672183, 99.43633196372844907, 4.000000000000000000 ) ) ;
#12012=CARTESIAN_POINT ( 'NONE',  ( 31.50000000000000711, 90.00000000000000000, 22.38477631085024555 ) ) ;
#12021=DIRECTION ( 'NONE',  ( 1.000000000000000000, -4.270088556250602685E-15, 0.000000000000000000 ) ) ;
#12067=( LENGTH_UNIT ( ) NAMED_UNIT ( * ) SI_UNIT ( .MILLI., .METRE. ) );
#12077=EDGE_CURVE ( 'NONE', #8914, #2081, #2773, .T. ) ;
#12092=ADVANCED_FACE ( 'NONE', ( #7735 ), #7542, .T. ) ;
#12095=ORIENTED_EDGE ( 'NONE', *, *, #3152, .T. ) ;
#12097=DIRECTION ( 'NONE',  ( -1.000000000000000000, 0.000000000000000000, 0.000000000000000000 ) ) ;
#12112=B_SPLINE_CURVE_WITH_KNOTS ( 'NONE', 3,
 ( #4737, #1726, #2716, #3892 ),
 .UNSPECIFIED., .F., .F.,
 ( 4, 4 ),
 ( 0.000000000000000000, 1.000000000000000000 ),
 .UNSPECIFIED. ) ;
#12130=DIRECTION ( 'NONE',  ( -1.000000000000000000, 0.000000000000000000, 0.000000000000000000 ) ) ;
#12141=EDGE_LOOP ( 'NONE', ( #9561, #5369, #2592, #10461 ) ) ;
#12144=EDGE_CURVE ( 'NONE', #7589, #11688, #238, .T. ) ;
#12149=ORIENTED_EDGE ( 'NONE', *, *, #913, .T. ) ;
#12158=DIRECTION ( 'NONE',  ( -0.000000000000000000, 0.000000000000000000, 1.000000000000000000 ) ) ;
#12161=CARTESIAN_POINT ( 'NONE',  ( 31.50000000000000711, 90.00000000000000000, 4.000000000000000000 ) ) ;
#12169=ORIENTED_EDGE ( 'NONE', *, *, #2930, .T. ) ;
#12180=VERTEX_POINT ( 'NONE', #4137 ) ;
#12196=FACE_OUTER_BOUND ( 'NONE', #5152, .T. ) ;
#12213=DIRECTION ( 'NONE',  ( 0.3090169943749492276, -0.9510565162951530871, 0.000000000000000000 ) ) ;
#12220=ORIENTED_EDGE ( 'NONE', *, *, #11469, .F. ) ;
#12222=DIRECTION ( 'NONE',  ( 0.000000000000000000, 0.000000000000000000, 1.000000000000000000 ) ) ;
#12228=ORIENTED_EDGE ( 'NONE', *, *, #6632, .T. ) ;
#12243=DIRECTION ( 'NONE',  ( -0.000000000000000000, -0.000000000000000000, -1.000000000000000000 ) ) ;
#12246=AXIS2_PLACEMENT_3D ( 'NONE', #12721, #7940, #5844 ) ;
#12255=ORIENTED_EDGE ( 'NONE', *, *, #7635, .F. ) ;
#12256=PRODUCT_DEFINITION ( 'UNKNOWN', '', #6348, #1232 ) ;
#12278=CARTESIAN_POINT ( 'NONE',  ( 41.00904217445252442, 92.47818727009297390, 4.000000000000000000 ) ) ;
#12295=ORIENTED_EDGE ( 'NONE', *, *, #8076, .T. ) ;
#12296=DIRECTION ( 'NONE',  ( 0.000000000000000000, -0.000000000000000000, 1.000000000000000000 ) ) ;
#12303=AXIS2_PLACEMENT_3D ( 'NONE', #5803, #8625, #10708 ) ;
#12307=CYLINDRICAL_SURFACE ( 'NONE', #12918, 6.499999999999999112 ) ;
#12309=VECTOR ( 'NONE', #3502, 1000.000000000000000 ) ;
#12318=VERTEX_POINT ( 'NONE', #6147 ) ;
#12333=DIRECTION ( 'NONE',  ( 0.000000000000000000, 0.000000000000000000, 1.000000000000000000 ) ) ;
#12337=CARTESIAN_POINT ( 'NONE',  ( 16.96438320935645905, 66.02675393316422969, -0.9999999999999970024 ) ) ;
#12338=ORIENTED_EDGE ( 'NONE', *, *, #11563, .F. ) ;
#12361=FACE_BOUND ( 'NONE', #4316, .T. ) ;
#12364=ORIENTED_EDGE ( 'NONE', *, *, #1518, .T. ) ;
#12385=LINE ( 'NONE', #1460, #7302 ) ;
#12389=DIRECTION ( 'NONE',  ( 1.000000000000000000, 0.000000000000000000, 0.000000000000000000 ) ) ;
#12399=VERTEX_POINT ( 'NONE', #10602 ) ;
#12405=ORIENTED_EDGE ( 'NONE', *, *, #3482, .F. ) ;
#12411=DIRECTION ( 'NONE',  ( 0.000000000000000000, 0.000000000000000000, 1.000000000000000000 ) ) ;
#12416=LINE ( 'NONE', #630, #11548 ) ;
#12444=CARTESIAN_POINT ( 'NONE',  ( -15.06519709809452756, 92.38262548349219117, 1.000000000000003109 ) ) ;
#12445=AXIS2_PLACEMENT_3D ( 'NONE', #2551, #12296, #6529 ) ;
#12463=CARTESIAN_POINT ( 'NONE',  ( 52.45028081366923089, 66.83239978927284142, 0.6666666666666665186 ) ) ;
#12464=PLANE ( 'NONE',  #11207 ) ;
#12465=ORIENTED_EDGE ( 'NONE', *, *, #6976, .F. ) ;
#12469=EDGE_LOOP ( 'NONE', ( #3320, #11981, #328, #2072, #355, #11371 ) ) ;
#12470=CIRCLE ( 'NONE', #3906, 6.499999999999999112 ) ;
#12499=ADVANCED_FACE ( 'NONE', ( #10000 ), #3076, .T. ) ;
#12517=CARTESIAN_POINT ( 'NONE',  ( 51.63935276957964504, 66.24642824321904300, 4.000000000000000000 ) ) ;
#12518=DIRECTION ( 'NONE',  ( 0.000000000000000000, 0.000000000000000000, -1.000000000000000000 ) ) ;
#12520=VECTOR ( 'NONE', #3153, 1000.000000000000000 ) ;
#12523=CARTESIAN_POINT ( 'NONE',  ( 12.55092940903992194, 109.9007343985615393, 1.000000000000003553 ) ) ;
#12525=CARTESIAN_POINT ( 'NONE',  ( 31.50000000000000711, 90.00000000000000000, -3.000000000000000000 ) ) ;
#12529=EDGE_CURVE ( 'NONE', #7127, #9471, #37, .T. ) ;
#12530=AXIS2_PLACEMENT_3D ( 'NONE', #3756, #11854, #7738 ) ;
#12534=LINE ( 'NONE', #4116, #10277 ) ;
#12536=ORIENTED_EDGE ( 'NONE', *, *, #6705, .T. ) ;
#12537=SURFACE_STYLE_FILL_AREA ( #10501 ) ;
#12541=APPLICATION_CONTEXT ( 'automotive_design' ) ;
#12561=DIRECTION ( 'NONE',  ( -0.9510565162951529761, -0.3090169943749492276, 0.000000000000000000 ) ) ;
#12571=ADVANCED_FACE ( 'NONE', ( #6926 ), #10910, .T. ) ;
#12572=ADVANCED_FACE ( 'NONE', ( #6988, #5085, #3006 ), #4118, .T. ) ;
#12583=DIRECTION ( 'NONE',  ( -0.3090169943749500048, 0.9510565162951528650, 0.000000000000000000 ) ) ;
#12590=DIRECTION ( 'NONE',  ( 0.000000000000000000, 0.000000000000000000, 1.000000000000000000 ) ) ;
#12600=EDGE_CURVE ( 'NONE', #6886, #7310, #4445, .T. ) ;
#12615=CIRCLE ( 'NONE', #1320, 28.99999999999999289 ) ;
#12619=( GEOMETRIC_REPRESENTATION_CONTEXT ( 3 ) GLOBAL_UNCERTAINTY_ASSIGNED_CONTEXT ( ( #9623 ) ) GLOBAL_UNIT_ASSIGNED_CONTEXT ( ( #10017, #6767, #2788 ) ) REPRESENTATION_CONTEXT ( 'NONE', 'WORKASPACE' ) );
#12638=CIRCLE ( 'NONE', #8037, 29.99999999999999645 ) ;
#12641=VERTEX_POINT ( 'NONE', #9142 ) ;
#12655=AXIS2_PLACEMENT_3D ( 'NONE', #7060, #11043, #12097 ) ;
#12656=DIRECTION ( 'NONE',  ( 0.8090169943749476733, 0.5877852522924726930, 0.000000000000000000 ) ) ;
#12657=LINE ( 'NONE', #4611, #10845 ) ;
#12664=ORIENTED_EDGE ( 'NONE', *, *, #12833, .F. ) ;
#12674=CARTESIAN_POINT ( 'NONE',  ( 51.64126381929429499, 66.24461453698036451, 4.000000000000000000 ) ) ;
#12679=EDGE_LOOP ( 'NONE', ( #1114, #7969, #6216, #8005 ) ) ;
#12708=VECTOR ( 'NONE', #8320, 1000.000000000000000 ) ;
#12709=DIRECTION ( 'NONE',  ( -0.000000000000000000, -0.000000000000000000, -1.000000000000000000 ) ) ;
#12721=CARTESIAN_POINT ( 'NONE',  ( 35.00000000000000000, 90.00000000000000000, 4.000000000000000000 ) ) ;
#12740=VECTOR ( 'NONE', #4400, 1000.000000000000114 ) ;
#12741=CARTESIAN_POINT ( 'NONE',  ( 62.42613047537196991, 99.43702109502110886, 0.6666666666666665186 ) ) ;
#12746=ADVANCED_FACE ( 'NONE', ( #10646 ), #1748, .F. ) ;
#12755=ORIENTED_EDGE ( 'NONE', *, *, #3830, .F. ) ;
#12780=PLANE ( 'NONE',  #2511 ) ;
#12781=DIRECTION ( 'NONE',  ( -1.000000000000000000, 0.000000000000000000, 0.000000000000000000 ) ) ;
#12806=FACE_OUTER_BOUND ( 'NONE', #11423, .T. ) ;
#12814=CYLINDRICAL_SURFACE ( 'NONE', #5261, 28.99999999999999289 ) ;
#12833=EDGE_CURVE ( 'NONE', #9167, #4318, #12416, .T. ) ;
#12837=DIRECTION ( 'NONE',  ( 0.000000000000000000, 0.000000000000000000, -1.000000000000000000 ) ) ;
#12841=CARTESIAN_POINT ( 'NONE',  ( 65.00000000000000000, 90.00000000000000000, -3.000000000000000000 ) ) ;
#12842=CARTESIAN_POINT ( 'NONE',  ( 13.95244456248789788, 109.9499476216067819, 4.000000000000000000 ) ) ;
#12843=ORIENTED_EDGE ( 'NONE', *, *, #7949, .T. ) ;
#12846=DIRECTION ( 'NONE',  ( -1.000000000000000000, 0.000000000000000000, 0.000000000000000000 ) ) ;
#12874=CARTESIAN_POINT ( 'NONE',  ( 72.83557806687970526, 62.54593364529978317, -0.9999999999999970024 ) ) ;
#12877=ORIENTED_EDGE ( 'NONE', *, *, #1839, .F. ) ;
#12880=DIRECTION ( 'NONE',  ( -0.000000000000000000, -0.000000000000000000, -1.000000000000000000 ) ) ;
#12892=VERTEX_POINT ( 'NONE', #10518 ) ;
#12918=AXIS2_PLACEMENT_3D ( 'NONE', #1750, #321, #7578 ) ;
#12923=PLANE ( 'NONE',  #8457 ) ;
#12941=VERTEX_POINT ( 'NONE', #5920 ) ;
#12945=EDGE_LOOP ( 'NONE', ( #11307, #4066, #9415, #4102 ) ) ;
#12946=AXIS2_PLACEMENT_3D ( 'NONE', #2453, #6426, #10425 ) ;
#13010=COLOUR_RGB('Off White',0.89,0.88,0.83);
#13011=FILL_AREA_STYLE_COLOUR('',#13010);
#13012=FILL_AREA_STYLE('',(#13011));
#13013=SURFACE_STYLE_FILL_AREA(#13012);
#13014=SURFACE_SIDE_STYLE('',(#13013));
#13015=SURFACE_STYLE_USAGE(.BOTH.,#13014);
#13016=PRESENTATION_STYLE_ASSIGNMENT((#13015));
ENDSEC;
END-ISO-10303-21;
